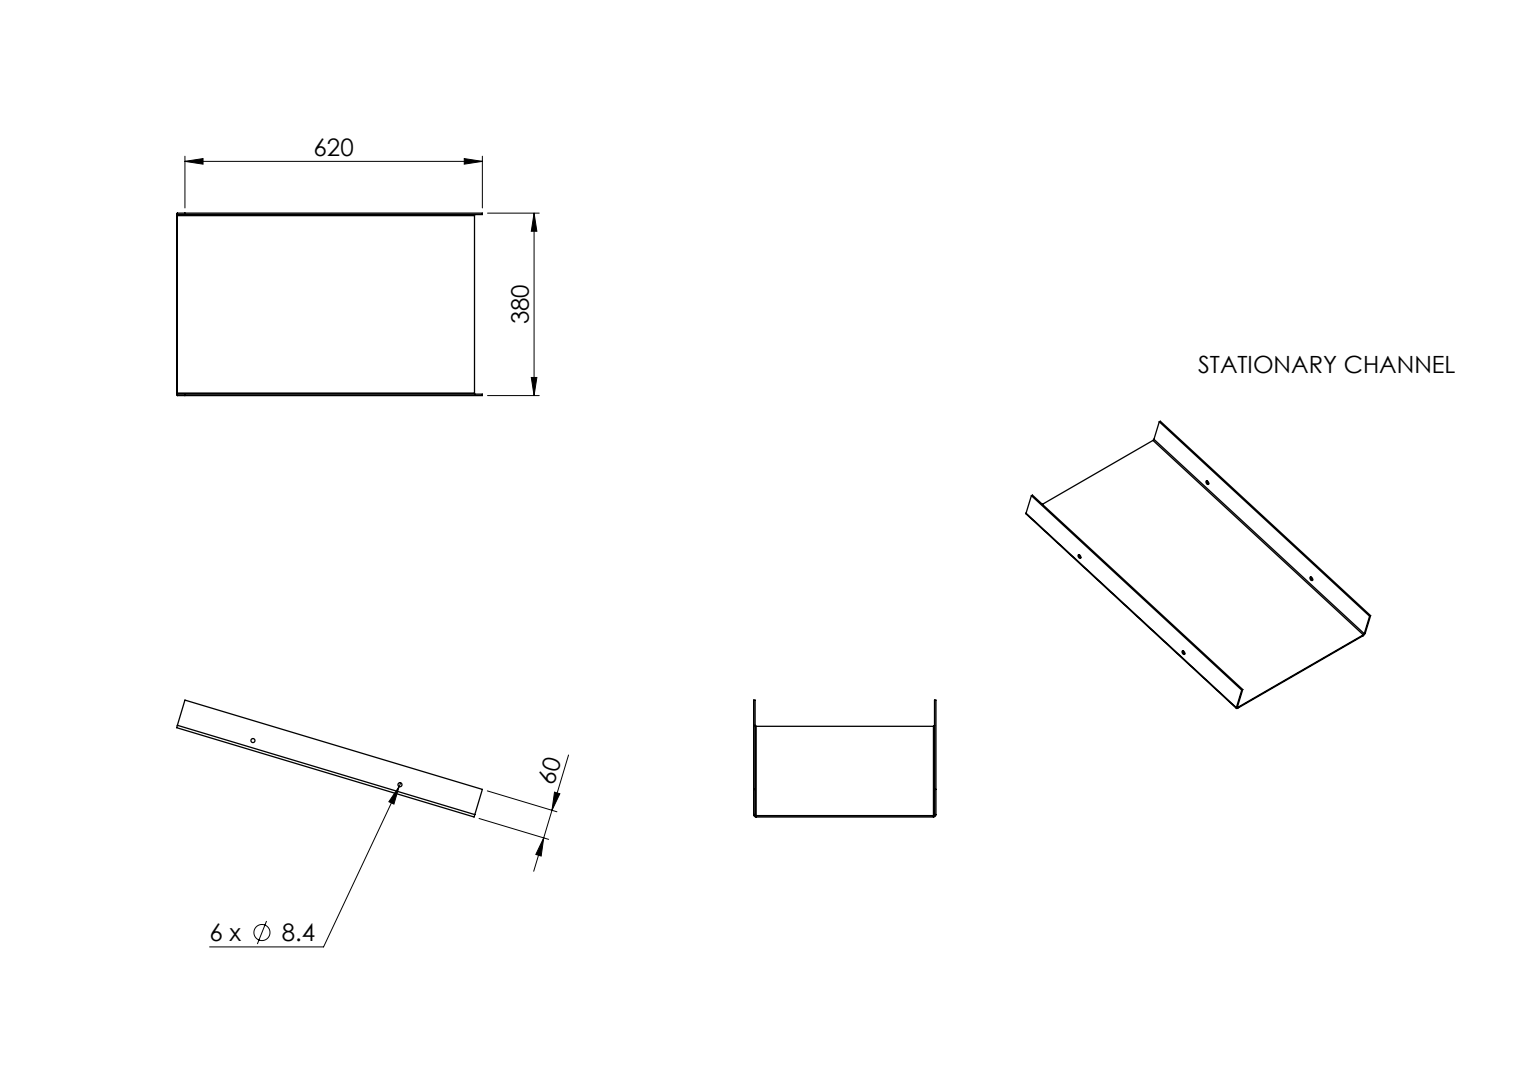
ISO-10303-21;
HEADER;
FILE_DESCRIPTION (('STEP AP214'),
    '1' );
FILE_NAME ('stationary channel.step',
    '2026-10-27T17:01:19',
    ( '' ),
    ( '' ),
    'SwSTEP 2.0',
    'SolidWorks 2026',
    '' );
FILE_SCHEMA (( 'AUTOMOTIVE_DESIGN' ));
ENDSEC;

DATA;
#27=FACE_OUTER_BOUND ( 'NONE', #636, .T. ) ;
#100=EDGE_LOOP ( 'NONE', ( #955, #2493 ) ) ;
#108=CARTESIAN_POINT ( 'NONE',  ( 610.0000000000000000, 227.4403065089097993, 184.7999999999999829 ) ) ;
#123=EDGE_CURVE ( 'NONE', #7138, #2816, #1501, .T. ) ;
#126=EDGE_CURVE ( 'NONE', #13510, #3531, #3853, .T. ) ;
#129=ORIENTED_EDGE ( 'NONE', *, *, #11764, .F. ) ;
#141=EDGE_CURVE ( 'NONE', #2225, #13547, #11826, .T. ) ;
#143=ORIENTED_EDGE ( 'NONE', *, *, #1858, .T. ) ;
#160=ADVANCED_FACE ( 'NONE', ( #9907 ), #3261, .F. ) ;
#164=ORIENTED_EDGE ( 'NONE', *, *, #10968, .F. ) ;
#185=PLANE ( 'NONE',  #4357 ) ;
#220=CIRCLE ( 'NONE', #10375, 2.199999999999988187 ) ;
#233=VECTOR ( 'NONE', #11079, 1000.000000000000000 ) ;
#245=CIRCLE ( 'NONE', #8768, 4.199999999999926459 ) ;
#249=DIRECTION ( 'NONE',  ( 0.9578262852211507639, -0.2873478855663477716, 0.000000000000000000 ) ) ;
#250=CARTESIAN_POINT ( 'NONE',  ( 153.1991633467111456, 386.6211705227183870, -210.0000000000000000 ) ) ;
#251=CARTESIAN_POINT ( 'NONE',  ( 627.2408731339806991, 284.9098836221797342, 190.0000000000001990 ) ) ;
#277=EDGE_LOOP ( 'NONE', ( #11682, #4913 ) ) ;
#280=LINE ( 'NONE', #3777, #11997 ) ;
#304=DIRECTION ( 'NONE',  ( 0.2873478855663427756, 0.9578262852211522071, 3.408579461568464094E-15 ) ) ;
#314=LINE ( 'NONE', #3891, #1590 ) ;
#379=VECTOR ( 'NONE', #7531, 1000.000000000000000 ) ;
#429=CARTESIAN_POINT ( 'NONE',  ( -8.505790995054768544, 418.4210031920615620, -184.7999999999999829 ) ) ;
#474=CARTESIAN_POINT ( 'NONE',  ( -9.137956343300835726, 416.3137853645748692, 184.7999999999999829 ) ) ;
#490=CARTESIAN_POINT ( 'NONE',  ( -1.861313246464723443E-13, -6.204377488215742287E-13, -186.9999999999986358 ) ) ;
#533=DIRECTION ( 'NONE',  ( -0.2873478855663454401, -0.9578262852211514300, -3.548540470164184620E-15 ) ) ;
#535=DIRECTION ( 'NONE',  ( -0.9578262852211513190, 0.2873478855663455511, 5.916456789157588541E-31 ) ) ;
#561=EDGE_CURVE ( 'NONE', #2165, #8693, #8490, .T. ) ;
#571=ORIENTED_EDGE ( 'NONE', *, *, #126, .T. ) ;
#576=DIRECTION ( 'NONE',  ( 0.9578262852211509859, -0.2873478855663466613, -4.622231866529364646E-30 ) ) ;
#588=DIRECTION ( 'NONE',  ( 9.794481010665704304E-16, 3.264827003555234768E-15, -1.000000000000000000 ) ) ;
#600=PLANE ( 'NONE',  #7043 ) ;
#605=ORIENTED_EDGE ( 'NONE', *, *, #2988, .F. ) ;
#610=LINE ( 'NONE', #474, #9375 ) ;
#626=DIRECTION ( 'NONE',  ( -0.9578262852211506528, 0.2873478855663477161, -0.000000000000000000 ) ) ;
#628=ORIENTED_EDGE ( 'NONE', *, *, #1225, .F. ) ;
#636=EDGE_LOOP ( 'NONE', ( #8796, #4569, #3020, #13957 ) ) ;
#679=CIRCLE ( 'NONE', #4453, 4.199999999999926459 ) ;
#681=VERTEX_POINT ( 'NONE', #2049 ) ;
#755=CARTESIAN_POINT ( 'NONE',  ( 153.1991633467111456, 386.6211705227183870, -190.0000000000000568 ) ) ;
#761=ORIENTED_EDGE ( 'NONE', *, *, #6990, .T. ) ;
#766=AXIS2_PLACEMENT_3D ( 'NONE', #3828, #7354, #8310 ) ;
#786=CARTESIAN_POINT ( 'NONE',  ( 451.3035746174797396, 294.6698471414878782, 190.0000000000000568 ) ) ;
#789=LINE ( 'NONE', #846, #1204 ) ;
#807=ADVANCED_FACE ( 'NONE', ( #7749 ), #14614, .F. ) ;
#812=ADVANCED_FACE ( 'NONE', ( #2126 ), #185, .T. ) ;
#820=DIRECTION ( 'NONE',  ( 0.000000000000000000, 1.000000000000000000, 0.000000000000000000 ) ) ;
#824=FACE_OUTER_BOUND ( 'NONE', #10572, .T. ) ;
#840=ORIENTED_EDGE ( 'NONE', *, *, #9284, .F. ) ;
#846=CARTESIAN_POINT ( 'NONE',  ( 610.8620436566989156, 230.3137853645742155, -187.0000000000000000 ) ) ;
#852=VERTEX_POINT ( 'NONE', #8038 ) ;
#858=DIRECTION ( 'NONE',  ( 0.2873478855663483267, 0.9578262852211505418, 0.000000000000000000 ) ) ;
#862=VECTOR ( 'NONE', #10859, 1000.000000000000114 ) ;
#863=CIRCLE ( 'NONE', #11005, 4.199999999999926459 ) ;
#868=DIRECTION ( 'NONE',  ( 1.921916333308140812E-15, 6.406387777693824270E-15, -1.000000000000000000 ) ) ;
#872=AXIS2_PLACEMENT_3D ( 'NONE', #1257, #4650, #7898 ) ;
#942=EDGE_CURVE ( 'NONE', #8737, #2165, #12678, .T. ) ;
#953=( GEOMETRIC_REPRESENTATION_CONTEXT ( 3 ) GLOBAL_UNCERTAINTY_ASSIGNED_CONTEXT ( ( #3993 ) ) GLOBAL_UNIT_ASSIGNED_CONTEXT ( ( #2035, #12214, #5452 ) ) REPRESENTATION_CONTEXT ( 'NONE', 'WORKASPACE' ) );
#955=ORIENTED_EDGE ( 'NONE', *, *, #1459, .T. ) ;
#958=DIRECTION ( 'NONE',  ( 0.000000000000000000, 1.000000000000000000, 3.264827003555234768E-15 ) ) ;
#985=ORIENTED_EDGE ( 'NONE', *, *, #1375, .T. ) ;
#995=AXIS2_PLACEMENT_3D ( 'NONE', #2091, #13260, #4330 ) ;
#1012=VERTEX_POINT ( 'NONE', #4251 ) ;
#1014=DIRECTION ( 'NONE',  ( 0.9578262852211507639, -0.2873478855663477716, 0.000000000000000000 ) ) ;
#1020=DIRECTION ( 'NONE',  ( -0.000000000000000000, -0.000000000000000000, -1.000000000000000000 ) ) ;
#1044=ADVANCED_FACE ( 'NONE', ( #2017 ), #14502, .F. ) ;
#1072=CARTESIAN_POINT ( 'NONE',  ( 455.5035746174796714, 294.6698471414878782, 187.0000000000000568 ) ) ;
#1131=ADVANCED_FACE ( 'NONE', ( #11459 ), #3428, .F. ) ;
#1141=AXIS2_PLACEMENT_3D ( 'NONE', #1241, #5744, #10241 ) ;
#1165=DIRECTION ( 'NONE',  ( 1.000000000000000000, 0.000000000000000000, 0.000000000000000000 ) ) ;
#1176=EDGE_LOOP ( 'NONE', ( #12389, #12490, #761, #12684 ) ) ;
#1178=CARTESIAN_POINT ( 'NONE',  ( 611.4942090049449916, 232.4210031920605388, 187.0000000000000000 ) ) ;
#1204=VECTOR ( 'NONE', #5366, 1000.000000000000227 ) ;
#1225=EDGE_CURVE ( 'NONE', #852, #13547, #7265, .T. ) ;
#1241=CARTESIAN_POINT ( 'NONE',  ( -8.505790995054995918, 418.4210031920614483, 184.7999999999999829 ) ) ;
#1247=AXIS2_PLACEMENT_3D ( 'NONE', #5486, #5271, #5189 ) ;
#1257=CARTESIAN_POINT ( 'NONE',  ( 611.4942090049451053, 232.4210031920599420, -184.7999999999999829 ) ) ;
#1274=CARTESIAN_POINT ( 'NONE',  ( 627.2408731339806991, 284.9098836221797342, 187.0000000000001990 ) ) ;
#1285=DIRECTION ( 'NONE',  ( -0.2873478855663483267, -0.9578262852211505418, -5.337610695313246651E-15 ) ) ;
#1318=DIRECTION ( 'NONE',  ( 0.9578262852211513190, -0.2873478855663453846, 0.000000000000000000 ) ) ;
#1333=EDGE_LOOP ( 'NONE', ( #7672, #14460, #2611, #6334 ) ) ;
#1344=LINE ( 'NONE', #4537, #4523 ) ;
#1347=EDGE_LOOP ( 'NONE', ( #7153, #12726, #8039, #8024 ) ) ;
#1354=DIRECTION ( 'NONE',  ( -0.2873478855663441633, -0.9578262852211516520, 3.408579461568462910E-15 ) ) ;
#1373=ORIENTED_EDGE ( 'NONE', *, *, #126, .F. ) ;
#1374=ADVANCED_FACE ( 'NONE', ( #4987 ), #9704, .F. ) ;
#1375=EDGE_CURVE ( 'NONE', #6946, #8693, #8587, .T. ) ;
#1376=VERTEX_POINT ( 'NONE', #755 ) ;
#1384=FACE_OUTER_BOUND ( 'NONE', #9975, .T. ) ;
#1390=CARTESIAN_POINT ( 'NONE',  ( 611.4942090049451053, 232.4210031920605388, 190.0000000000000000 ) ) ;
#1423=VECTOR ( 'NONE', #7760, 1000.000000000000000 ) ;
#1434=DIRECTION ( 'NONE',  ( -0.000000000000000000, -0.000000000000000000, 1.000000000000000000 ) ) ;
#1448=CIRCLE ( 'NONE', #1920, 4.199999999999926459 ) ;
#1459=EDGE_CURVE ( 'NONE', #10035, #14129, #8436, .T. ) ;
#1460=EDGE_LOOP ( 'NONE', ( #10013, #14172, #4888, #11929 ) ) ;
#1501=LINE ( 'NONE', #12864, #2181 ) ;
#1504=EDGE_CURVE ( 'NONE', #6153, #7939, #11006, .T. ) ;
#1516=LINE ( 'NONE', #9412, #9511 ) ;
#1526=EDGE_CURVE ( 'NONE', #10480, #13545, #3745, .T. ) ;
#1546=DIRECTION ( 'NONE',  ( -0.9578262852211507639, 0.2873478855663477716, -0.000000000000000000 ) ) ;
#1548=PLANE ( 'NONE',  #11567 ) ;
#1552=LINE ( 'NONE', #10711, #12900 ) ;
#1584=CARTESIAN_POINT ( 'NONE',  ( 611.4942090049448780, 232.4210031920598283, 184.7999999999999829 ) ) ;
#1590=VECTOR ( 'NONE', #9416, 1000.000000000000000 ) ;
#1592=VECTOR ( 'NONE', #10818, 1000.000000000000114 ) ;
#1596=DIRECTION ( 'NONE',  ( -0.000000000000000000, -0.000000000000000000, -1.000000000000000000 ) ) ;
#1618=FACE_BOUND ( 'NONE', #5385, .T. ) ;
#1633=FACE_BOUND ( 'NONE', #13457, .T. ) ;
#1648=DIRECTION ( 'NONE',  ( -0.2873478855663427756, -0.9578262852211522071, 0.000000000000000000 ) ) ;
#1702=AXIS2_PLACEMENT_3D ( 'NONE', #4505, #4645, #1165 ) ;
#1718=PLANE ( 'NONE',  #13443 ) ;
#1726=EDGE_CURVE ( 'NONE', #9048, #852, #1552, .T. ) ;
#1728=DIRECTION ( 'NONE',  ( 9.794481010665704304E-16, 3.264827003555234768E-15, -1.000000000000000000 ) ) ;
#1748=EDGE_CURVE ( 'NONE', #6946, #6153, #12852, .T. ) ;
#1756=ORIENTED_EDGE ( 'NONE', *, *, #1901, .F. ) ;
#1768=EDGE_LOOP ( 'NONE', ( #1792, #14548 ) ) ;
#1777=CARTESIAN_POINT ( 'NONE',  ( -10.00000000000007105, 413.4403065089107372, 184.7999999999999829 ) ) ;
#1792=ORIENTED_EDGE ( 'NONE', *, *, #10146, .T. ) ;
#1796=CARTESIAN_POINT ( 'NONE',  ( 610.8620436566991430, 230.3137853645733912, -184.7999999999999829 ) ) ;
#1802=LINE ( 'NONE', #11845, #13199 ) ;
#1847=CARTESIAN_POINT ( 'NONE',  ( 611.4942090049448780, 232.4210031920598283, 187.0000000000000000 ) ) ;
#1858=EDGE_CURVE ( 'NONE', #5524, #13510, #8711, .T. ) ;
#1869=EDGE_LOOP ( 'NONE', ( #5841, #9339, #9809, #5523 ) ) ;
#1870=ADVANCED_FACE ( 'NONE', ( #13141 ), #5390, .T. ) ;
#1901=EDGE_CURVE ( 'NONE', #4077, #8268, #9755, .T. ) ;
#1904=PRESENTATION_STYLE_ASSIGNMENT (( #3013 ) ) ;
#1912=VERTEX_POINT ( 'NONE', #14396 ) ;
#1916=DIRECTION ( 'NONE',  ( -0.000000000000000000, -0.000000000000000000, -1.000000000000000000 ) ) ;
#1920=AXIS2_PLACEMENT_3D ( 'NONE', #3888, #7564, #11017 ) ;
#1933=ADVANCED_FACE ( 'NONE', ( #6571 ), #14256, .F. ) ;
#1940=ORIENTED_EDGE ( 'NONE', *, *, #5847, .F. ) ;
#1961=LINE ( 'NONE', #10363, #9746 ) ;
#1966=EDGE_CURVE ( 'NONE', #7989, #9048, #9818, .T. ) ;
#1981=CARTESIAN_POINT ( 'NONE',  ( 611.4942090049451053, 232.4210031920599135, -187.0000000000000000 ) ) ;
#1987=DIRECTION ( 'NONE',  ( -1.000000000000000000, 0.000000000000000000, 0.000000000000000000 ) ) ;
#2007=CARTESIAN_POINT ( 'NONE',  ( 627.2408731339805854, 284.9098836221799615, -190.0000000000001990 ) ) ;
#2017=FACE_OUTER_BOUND ( 'NONE', #1333, .T. ) ;
#2027=EDGE_CURVE ( 'NONE', #4077, #13098, #3961, .T. ) ;
#2035=( LENGTH_UNIT ( ) NAMED_UNIT ( * ) SI_UNIT ( .MILLI., .METRE. ) );
#2041=ADVANCED_FACE ( 'NONE', ( #3327 ), #8042, .T. ) ;
#2044=AXIS2_PLACEMENT_3D ( 'NONE', #7770, #12258, #820 ) ;
#2049=CARTESIAN_POINT ( 'NONE',  ( 610.8620436566989156, 230.3137853645732775, 184.7999999999999829 ) ) ;
#2055=DIRECTION ( 'NONE',  ( 0.000000000000000000, -1.000000000000000000, 0.000000000000000000 ) ) ;
#2065=AXIS2_PLACEMENT_3D ( 'NONE', #9984, #3195, #2069 ) ;
#2069=DIRECTION ( 'NONE',  ( 0.000000000000000000, -1.000000000000000000, 0.000000000000000000 ) ) ;
#2091=CARTESIAN_POINT ( 'NONE',  ( 148.9991633467111569, 386.6211705227183870, -187.0000000000000568 ) ) ;
#2096=CARTESIAN_POINT ( 'NONE',  ( -8.505790995054976378, 418.4210031920615052, 190.0000000000000000 ) ) ;
#2107=DIRECTION ( 'NONE',  ( -0.2873478855663396114, -0.9578262852211530953, 0.000000000000000000 ) ) ;
#2125=VECTOR ( 'NONE', #7691, 1000.000000000000000 ) ;
#2126=FACE_OUTER_BOUND ( 'NONE', #7480, .T. ) ;
#2143=AXIS2_PLACEMENT_3D ( 'NONE', #9097, #2226, #2158 ) ;
#2149=ORIENTED_EDGE ( 'NONE', *, *, #13921, .T. ) ;
#2154=CIRCLE ( 'NONE', #12535, 2.199999999999988187 ) ;
#2158=DIRECTION ( 'NONE',  ( -1.000000000000000000, 0.000000000000000000, 0.000000000000000000 ) ) ;
#2165=VERTEX_POINT ( 'NONE', #10406 ) ;
#2181=VECTOR ( 'NONE', #8424, 1000.000000000000000 ) ;
#2198=FACE_BOUND ( 'NONE', #8661, .T. ) ;
#2201=FACE_OUTER_BOUND ( 'NONE', #14284, .T. ) ;
#2220=ORIENTED_EDGE ( 'NONE', *, *, #11012, .T. ) ;
#2225=VERTEX_POINT ( 'NONE', #1981 ) ;
#2226=DIRECTION ( 'NONE',  ( -0.000000000000000000, -0.000000000000000000, -1.000000000000000000 ) ) ;
#2248=SHAPE_REPRESENTATION ( 'stationary channel', ( #9440 ), #8508 ) ;
#2274=ORIENTED_EDGE ( 'NONE', *, *, #942, .T. ) ;
#2275=ORIENTED_EDGE ( 'NONE', *, *, #9049, .T. ) ;
#2288=EDGE_CURVE ( 'NONE', #12648, #9517, #610, .T. ) ;
#2304=DIRECTION ( 'NONE',  ( -0.000000000000000000, -0.000000000000000000, 1.000000000000000000 ) ) ;
#2307=EDGE_CURVE ( 'NONE', #10292, #10447, #314, .T. ) ;
#2320=VECTOR ( 'NONE', #13632, 1000.000000000000227 ) ;
#2325=CARTESIAN_POINT ( 'NONE',  ( -122.9652219749294488, 36.88956659247806869, -189.9999999999986358 ) ) ;
#2342=PLANE ( 'NONE',  #11572 ) ;
#2348=CARTESIAN_POINT ( 'NONE',  ( 112.9652219749295483, 376.5507399164318372, 1.650218294979717018E-14 ) ) ;
#2350=DIRECTION ( 'NONE',  ( -0.2873478855663477716, -0.9578262852211506528, 0.000000000000000000 ) ) ;
#2406=DIRECTION ( 'NONE',  ( -9.794481010665704304E-16, -3.264827003555233190E-15, -1.000000000000000000 ) ) ;
#2413=DIRECTION ( 'NONE',  ( 0.2873478855663448850, 0.9578262852211515410, -3.408579461568462910E-15 ) ) ;
#2416=VECTOR ( 'NONE', #6630, 1000.000000000000000 ) ;
#2424=( GEOMETRIC_REPRESENTATION_CONTEXT ( 3 ) GLOBAL_UNCERTAINTY_ASSIGNED_CONTEXT ( ( #13447 ) ) GLOBAL_UNIT_ASSIGNED_CONTEXT ( ( #2705, #7205, #13845 ) ) REPRESENTATION_CONTEXT ( 'NONE', 'WORKASPACE' ) );
#2428=DIRECTION ( 'NONE',  ( 0.2873478855663454401, 0.9578262852211513190, 0.000000000000000000 ) ) ;
#2438=ORIENTED_EDGE ( 'NONE', *, *, #10439, .T. ) ;
#2493=ORIENTED_EDGE ( 'NONE', *, *, #12109, .T. ) ;
#2500=VERTEX_POINT ( 'NONE', #1847 ) ;
#2505=PRODUCT_DEFINITION_SHAPE ( 'NONE', 'NONE',  #5588 ) ;
#2524=AXIS2_PLACEMENT_3D ( 'NONE', #14594, #3384, #7942 ) ;
#2549=AXIS2_PLACEMENT_3D ( 'NONE', #12721, #11396, #1285 ) ;
#2589=LINE ( 'NONE', #3410, #5681 ) ;
#2611=ORIENTED_EDGE ( 'NONE', *, *, #123, .T. ) ;
#2631=CIRCLE ( 'NONE', #12512, 4.199999999999981526 ) ;
#2661=ORIENTED_EDGE ( 'NONE', *, *, #1966, .F. ) ;
#2665=LINE ( 'NONE', #6881, #11080 ) ;
#2672=CARTESIAN_POINT ( 'NONE',  ( 497.0347780250717733, -149.1104334075207589, 189.9999999999986358 ) ) ;
#2705=( LENGTH_UNIT ( ) NAMED_UNIT ( * ) SI_UNIT ( .MILLI., .METRE. ) );
#2744=ORIENTED_EDGE ( 'NONE', *, *, #2027, .F. ) ;
#2745=DIRECTION ( 'NONE',  ( -0.2873478855663480491, -0.9578262852211507639, 0.000000000000000000 ) ) ;
#2782=CYLINDRICAL_SURFACE ( 'NONE', #3577, 4.199999999999981526 ) ;
#2793=ORIENTED_EDGE ( 'NONE', *, *, #9284, .T. ) ;
#2816=VERTEX_POINT ( 'NONE', #8845 ) ;
#2827=LINE ( 'NONE', #13427, #5208 ) ;
#2833=EDGE_CURVE ( 'NONE', #6946, #8674, #3743, .T. ) ;
#2852=CYLINDRICAL_SURFACE ( 'NONE', #766, 2.200000000000007283 ) ;
#2865=LINE ( 'NONE', #3837, #14610 ) ;
#2894=ORIENTED_EDGE ( 'NONE', *, *, #14304, .T. ) ;
#2902=VERTEX_POINT ( 'NONE', #11482 ) ;
#2913=CARTESIAN_POINT ( 'NONE',  ( 627.2408731339806991, 284.9098836221797342, 190.0000000000001990 ) ) ;
#2929=CARTESIAN_POINT ( 'NONE',  ( -122.9652219749301736, 36.88956659247854475, 189.9999999999986358 ) ) ;
#2943=( NAMED_UNIT ( * ) SI_UNIT ( $, .STERADIAN. ) SOLID_ANGLE_UNIT ( ) );
#2960=DIRECTION ( 'NONE',  ( -0.2873478855663454401, -0.9578262852211513190, 0.000000000000000000 ) ) ;
#2977=CARTESIAN_POINT ( 'NONE',  ( 455.5035746174796714, 294.6698471414878782, 190.0000000000000568 ) ) ;
#2984=ORIENTED_EDGE ( 'NONE', *, *, #3700, .T. ) ;
#2988=EDGE_CURVE ( 'NONE', #9517, #8693, #12207, .T. ) ;
#3002=EDGE_CURVE ( 'NONE', #10447, #9874, #8027, .T. ) ;
#3013=SURFACE_STYLE_USAGE ( .BOTH. , #13122 ) ;
#3020=ORIENTED_EDGE ( 'NONE', *, *, #5314, .T. ) ;
#3026=CARTESIAN_POINT ( 'NONE',  ( 7.240873133980807452, 470.9098836221798479, -190.0000000000001990 ) ) ;
#3032=CARTESIAN_POINT ( 'NONE',  ( 459.7035746174795463, 294.6698471414878782, 210.0000000000000000 ) ) ;
#3035=ADVANCED_FACE ( 'NONE', ( #11563, #8540, #12971 ), #9923, .T. ) ;
#3038=ORIENTED_EDGE ( 'NONE', *, *, #10054, .T. ) ;
#3050=ORIENTED_EDGE ( 'NONE', *, *, #6990, .F. ) ;
#3052=DIRECTION ( 'NONE',  ( -0.2873478855663441633, -0.9578262852211516520, 0.000000000000000000 ) ) ;
#3088=STYLED_ITEM ( 'NONE', ( #1904 ), #12520 ) ;
#3101=DIRECTION ( 'NONE',  ( 0.000000000000000000, -1.000000000000000000, 3.264827003555233190E-15 ) ) ;
#3167=( NAMED_UNIT ( * ) PLANE_ANGLE_UNIT ( ) SI_UNIT ( $, .RADIAN. ) );
#3194=ORIENTED_EDGE ( 'NONE', *, *, #6816, .T. ) ;
#3195=DIRECTION ( 'NONE',  ( -9.794481010665704304E-16, -3.264827003555233190E-15, -1.000000000000000000 ) ) ;
#3223=VERTEX_POINT ( 'NONE', #3421 ) ;
#3228=SHAPE_REPRESENTATION_RELATIONSHIP ( 'NONE' , 'NONE' ,  #2248, #12520 ) ;
#3233=CARTESIAN_POINT ( 'NONE',  ( 611.4942090049448780, 232.4210031920598283, 184.7999999999999829 ) ) ;
#3261=PLANE ( 'NONE',  #1247 ) ;
#3270=AXIS2_PLACEMENT_3D ( 'NONE', #12259, #6671, #4530 ) ;
#3276=ORIENTED_EDGE ( 'NONE', *, *, #8006, .T. ) ;
#3298=EDGE_LOOP ( 'NONE', ( #3194, #14214 ) ) ;
#3299=DIRECTION ( 'NONE',  ( 0.000000000000000000, 1.000000000000000000, 0.000000000000000000 ) ) ;
#3327=FACE_OUTER_BOUND ( 'NONE', #14566, .T. ) ;
#3344=LINE ( 'NONE', #5545, #2125 ) ;
#3351=CIRCLE ( 'NONE', #7344, 2.200000000000009948 ) ;
#3384=DIRECTION ( 'NONE',  ( -0.9578262852211507639, 0.2873478855663477716, 0.000000000000000000 ) ) ;
#3406=DIRECTION ( 'NONE',  ( -0.9578262852211507639, 0.2873478855663477716, 0.000000000000000000 ) ) ;
#3410=CARTESIAN_POINT ( 'NONE',  ( -9.999999999999840128, 413.4403065089115330, -184.7999999999999829 ) ) ;
#3421=CARTESIAN_POINT ( 'NONE',  ( 144.7991633467111683, 386.6211705227183870, 190.0000000000000568 ) ) ;
#3422=DIRECTION ( 'NONE',  ( 0.2873478855663477161, 0.9578262852211506528, 0.000000000000000000 ) ) ;
#3428=CYLINDRICAL_SURFACE ( 'NONE', #4683, 4.199999999999926459 ) ;
#3443=CYLINDRICAL_SURFACE ( 'NONE', #2524, 2.200000000000007283 ) ;
#3450=ORIENTED_EDGE ( 'NONE', *, *, #12173, .F. ) ;
#3462=LINE ( 'NONE', #11427, #6116 ) ;
#3502=VERTEX_POINT ( 'NONE', #7543 ) ;
#3506=VECTOR ( 'NONE', #11881, 1000.000000000000114 ) ;
#3531=VERTEX_POINT ( 'NONE', #9693 ) ;
#3547=ORIENTED_EDGE ( 'NONE', *, *, #10808, .F. ) ;
#3573=FACE_OUTER_BOUND ( 'NONE', #6762, .T. ) ;
#3577=AXIS2_PLACEMENT_3D ( 'NONE', #12000, #1596, #7364 ) ;
#3588=FACE_OUTER_BOUND ( 'NONE', #6490, .T. ) ;
#3619=CARTESIAN_POINT ( 'NONE',  ( 148.9991633467111569, 386.6211705227183870, 187.0000000000000568 ) ) ;
#3626=CARTESIAN_POINT ( 'NONE',  ( 451.3035746174797396, 294.6698471414878782, 187.0000000000000568 ) ) ;
#3668=DIRECTION ( 'NONE',  ( 0.9578262852211513190, -0.2873478855663453846, 0.000000000000000000 ) ) ;
#3677=ORIENTED_EDGE ( 'NONE', *, *, #13247, .F. ) ;
#3700=EDGE_CURVE ( 'NONE', #9517, #3531, #280, .T. ) ;
#3743=CIRCLE ( 'NONE', #13633, 5.200000000000005507 ) ;
#3745=CIRCLE ( 'NONE', #2044, 4.199999999999981526 ) ;
#3757=ORIENTED_EDGE ( 'NONE', *, *, #141, .T. ) ;
#3777=CARTESIAN_POINT ( 'NONE',  ( -9.999999999999980460, 413.4403065089106235, 190.0000000000000000 ) ) ;
#3790=VECTOR ( 'NONE', #9846, 1000.000000000000000 ) ;
#3828=CARTESIAN_POINT ( 'NONE',  ( 611.4942090049449916, 232.4210031920597999, 184.7999999999999829 ) ) ;
#3837=CARTESIAN_POINT ( 'NONE',  ( 610.8620436566990293, 230.3137853645732491, 184.7999999999999829 ) ) ;
#3850=ORIENTED_EDGE ( 'NONE', *, *, #14304, .F. ) ;
#3853=CIRCLE ( 'NONE', #5726, 5.200000000000004619 ) ;
#3888=CARTESIAN_POINT ( 'NONE',  ( 455.5035746174796714, 294.6698471414878782, -190.0000000000000568 ) ) ;
#3891=CARTESIAN_POINT ( 'NONE',  ( 7.240873133980807452, 470.9098836221799047, -190.0000000000001990 ) ) ;
#3893=CARTESIAN_POINT ( 'NONE',  ( 459.7035746174795463, 294.6698471414878782, -210.0000000000000000 ) ) ;
#3894=DIRECTION ( 'NONE',  ( -0.000000000000000000, -0.000000000000000000, -1.000000000000000000 ) ) ;
#3909=DIRECTION ( 'NONE',  ( 0.000000000000000000, -1.000000000000000000, 0.000000000000000000 ) ) ;
#3920=ADVANCED_FACE ( 'NONE', ( #1618, #7521, #3987 ), #12915, .F. ) ;
#3924=DIRECTION ( 'NONE',  ( -0.2873478855663894049, -0.9578262852211382183, 0.000000000000000000 ) ) ;
#3948=ADVANCED_FACE ( 'NONE', ( #2198, #4417, #13344 ), #6562, .F. ) ;
#3955=DIRECTION ( 'NONE',  ( 0.000000000000000000, -5.337610695313242707E-15, 1.000000000000000000 ) ) ;
#3961=CIRCLE ( 'NONE', #11019, 4.199999999999926459 ) ;
#3971=CARTESIAN_POINT ( 'NONE',  ( -8.505790995054773873, 418.4210031920615620, -187.0000000000000000 ) ) ;
#3987=FACE_OUTER_BOUND ( 'NONE', #13183, .T. ) ;
#3993=UNCERTAINTY_MEASURE_WITH_UNIT (LENGTH_MEASURE( 1.000000000000000082E-05 ), #2035, 'distance_accuracy_value', 'NONE');
#4024=ORIENTED_EDGE ( 'NONE', *, *, #8205, .F. ) ;
#4036=CARTESIAN_POINT ( 'NONE',  ( 153.1991633467111456, 386.6211705227183870, 190.0000000000000568 ) ) ;
#4062=AXIS2_PLACEMENT_3D ( 'NONE', #13779, #4922, #3668 ) ;
#4077=VERTEX_POINT ( 'NONE', #11202 ) ;
#4085=VERTEX_POINT ( 'NONE', #14387 ) ;
#4101=DIRECTION ( 'NONE',  ( -0.9578262852211522071, 0.2873478855663427756, -9.629649721936179265E-30 ) ) ;
#4119=DIRECTION ( 'NONE',  ( 9.794481010665704304E-16, 3.264827003555234768E-15, -1.000000000000000000 ) ) ;
#4155=DIRECTION ( 'NONE',  ( -0.9578262852211513190, 0.2873478855663453846, 0.000000000000000000 ) ) ;
#4203=AXIS2_PLACEMENT_3D ( 'NONE', #8824, #8470, #8883 ) ;
#4232=EDGE_CURVE ( 'NONE', #681, #12648, #2865, .T. ) ;
#4251=CARTESIAN_POINT ( 'NONE',  ( 459.7035746174795463, 294.6698471414878782, -190.0000000000000568 ) ) ;
#4330=DIRECTION ( 'NONE',  ( 0.000000000000000000, -1.000000000000000000, 0.000000000000000000 ) ) ;
#4346=LINE ( 'NONE', #7593, #2416 ) ;
#4347=CARTESIAN_POINT ( 'NONE',  ( 0.000000000000000000, 0.000000000000000000, 0.000000000000000000 ) ) ;
#4357=AXIS2_PLACEMENT_3D ( 'NONE', #2348, #5533, #1318 ) ;
#4367=ORIENTED_EDGE ( 'NONE', *, *, #1726, .F. ) ;
#4380=EDGE_LOOP ( 'NONE', ( #3757, #3450, #5668, #10845 ) ) ;
#4396=ORIENTED_EDGE ( 'NONE', *, *, #7209, .T. ) ;
#4399=ORIENTED_EDGE ( 'NONE', *, *, #11764, .T. ) ;
#4417=FACE_BOUND ( 'NONE', #277, .T. ) ;
#4453=AXIS2_PLACEMENT_3D ( 'NONE', #9724, #4119, #11992 ) ;
#4461=AXIS2_PLACEMENT_3D ( 'NONE', #13419, #10023, #3101 ) ;
#4505=CARTESIAN_POINT ( 'NONE',  ( 148.9991633467111569, 386.6211705227183870, 210.0000000000000000 ) ) ;
#4520=FACE_OUTER_BOUND ( 'NONE', #1347, .T. ) ;
#4523=VECTOR ( 'NONE', #8951, 1000.000000000000000 ) ;
#4530=DIRECTION ( 'NONE',  ( 0.000000000000000000, 1.000000000000000000, 0.000000000000000000 ) ) ;
#4537=CARTESIAN_POINT ( 'NONE',  ( 451.3035746174797396, 294.6698471414878782, 210.0000000000000000 ) ) ;
#4549=CARTESIAN_POINT ( 'NONE',  ( 455.5035746174796714, 294.6698471414878782, 210.0000000000000000 ) ) ;
#4569=ORIENTED_EDGE ( 'NONE', *, *, #11840, .T. ) ;
#4577=DIRECTION ( 'NONE',  ( 9.794481010665704304E-16, 3.264827003555234768E-15, -1.000000000000000000 ) ) ;
#4641=CARTESIAN_POINT ( 'NONE',  ( 627.2408731339805854, 284.9098836221799615, -187.0000000000001990 ) ) ;
#4644=FACE_OUTER_BOUND ( 'NONE', #12280, .T. ) ;
#4645=DIRECTION ( 'NONE',  ( -0.000000000000000000, -0.000000000000000000, 1.000000000000000000 ) ) ;
#4650=DIRECTION ( 'NONE',  ( 0.9578262852211507639, -0.2873478855663477716, -0.000000000000000000 ) ) ;
#4669=EDGE_LOOP ( 'NONE', ( #2744, #3547 ) ) ;
#4675=ORIENTED_EDGE ( 'NONE', *, *, #4232, .F. ) ;
#4683=AXIS2_PLACEMENT_3D ( 'NONE', #13828, #1434, #10286 ) ;
#4707=ORIENTED_EDGE ( 'NONE', *, *, #10439, .F. ) ;
#4726=DIRECTION ( 'NONE',  ( 0.9578262852211514300, -0.2873478855663454956, 0.000000000000000000 ) ) ;
#4768=EDGE_CURVE ( 'NONE', #10480, #3223, #1516, .T. ) ;
#4796=CARTESIAN_POINT ( 'NONE',  ( -8.505790995055013681, 418.4210031920606525, 187.0000000000000000 ) ) ;
#4811=CARTESIAN_POINT ( 'NONE',  ( 610.8620436566989156, 230.3137853645732775, 184.7999999999999829 ) ) ;
#4815=ORIENTED_EDGE ( 'NONE', *, *, #942, .F. ) ;
#4847=EDGE_CURVE ( 'NONE', #5524, #10447, #8525, .T. ) ;
#4880=ORIENTED_EDGE ( 'NONE', *, *, #1526, .T. ) ;
#4888=ORIENTED_EDGE ( 'NONE', *, *, #2307, .F. ) ;
#4902=VECTOR ( 'NONE', #6314, 1000.000000000000114 ) ;
#4913=ORIENTED_EDGE ( 'NONE', *, *, #10628, .T. ) ;
#4922=DIRECTION ( 'NONE',  ( -0.2873478855663454401, -0.9578262852211514300, -4.197634718856730240E-17 ) ) ;
#4978=CIRCLE ( 'NONE', #13216, 4.199999999999981526 ) ;
#4987=FACE_OUTER_BOUND ( 'NONE', #11240, .T. ) ;
#5004=DIRECTION ( 'NONE',  ( -0.2873478855662898734, -0.9578262852211680833, 0.000000000000000000 ) ) ;
#5039=ADVANCED_FACE ( 'NONE', ( #5710 ), #1548, .F. ) ;
#5075=FACE_OUTER_BOUND ( 'NONE', #11435, .T. ) ;
#5101=DIRECTION ( 'NONE',  ( 0.000000000000000000, -1.000000000000000000, 0.000000000000000000 ) ) ;
#5132=ADVANCED_FACE ( 'NONE', ( #11933 ), #9814, .F. ) ;
#5140=LINE ( 'NONE', #8531, #4902 ) ;
#5142=ADVANCED_FACE ( 'NONE', ( #9593 ), #9750, .F. ) ;
#5152=ORIENTED_EDGE ( 'NONE', *, *, #9828, .T. ) ;
#5168=AXIS2_PLACEMENT_3D ( 'NONE', #2977, #1728, #13023 ) ;
#5178=CARTESIAN_POINT ( 'NONE',  ( 459.7035746174795463, 294.6698471414878782, 190.0000000000000568 ) ) ;
#5180=ORIENTED_EDGE ( 'NONE', *, *, #3002, .F. ) ;
#5189=DIRECTION ( 'NONE',  ( -0.2873478855663477161, -0.9578262852211506528, 0.000000000000000000 ) ) ;
#5208=VECTOR ( 'NONE', #1020, 1000.000000000000000 ) ;
#5254=DIRECTION ( 'NONE',  ( 0.000000000000000000, 1.000000000000000000, 0.000000000000000000 ) ) ;
#5258=DIRECTION ( 'NONE',  ( 0.2873478855663448850, 0.9578262852211515410, 0.000000000000000000 ) ) ;
#5271=DIRECTION ( 'NONE',  ( -0.9578262852211507639, 0.2873478855663477716, 0.000000000000000000 ) ) ;
#5291=LINE ( 'NONE', #2929, #1592 ) ;
#5314=EDGE_CURVE ( 'NONE', #2225, #5524, #13857, .T. ) ;
#5322=CARTESIAN_POINT ( 'NONE',  ( -9.137956343300796647, 416.3137853645750397, -184.7999999999999829 ) ) ;
#5366=DIRECTION ( 'NONE',  ( -0.2873478855663441633, -0.9578262852211516520, 3.408579461568462910E-15 ) ) ;
#5385=EDGE_LOOP ( 'NONE', ( #7964, #2438 ) ) ;
#5390=PLANE ( 'NONE',  #8203 ) ;
#5414=VERTEX_POINT ( 'NONE', #786 ) ;
#5423=ADVANCED_FACE ( 'NONE', ( #7434 ), #2782, .F. ) ;
#5452=( NAMED_UNIT ( * ) SI_UNIT ( $, .STERADIAN. ) SOLID_ANGLE_UNIT ( ) );
#5470=DIRECTION ( 'NONE',  ( -0.9578262852211514300, 0.2873478855663454956, -1.399211572952243085E-16 ) ) ;
#5485=CIRCLE ( 'NONE', #995, 4.199999999999981526 ) ;
#5486=CARTESIAN_POINT ( 'NONE',  ( 611.4942090049448780, 232.4210031920598283, 184.7999999999999829 ) ) ;
#5510=ORIENTED_EDGE ( 'NONE', *, *, #141, .F. ) ;
#5521=DIRECTION ( 'NONE',  ( 0.9578262852211507639, -0.2873478855663477716, -0.000000000000000000 ) ) ;
#5523=ORIENTED_EDGE ( 'NONE', *, *, #12173, .T. ) ;
#5524=VERTEX_POINT ( 'NONE', #3971 ) ;
#5533=DIRECTION ( 'NONE',  ( -0.2873478855663454401, -0.9578262852211514300, -4.197634718856730240E-17 ) ) ;
#5535=CARTESIAN_POINT ( 'NONE',  ( -9.137956343300944084, 416.3137853645740734, 190.0000000000000000 ) ) ;
#5545=CARTESIAN_POINT ( 'NONE',  ( -9.137956343300944084, 416.3137853645740734, 190.0000000000000000 ) ) ;
#5566=CYLINDRICAL_SURFACE ( 'NONE', #7145, 4.199999999999926459 ) ;
#5585=LINE ( 'NONE', #4796, #12004 ) ;
#5588=PRODUCT_DEFINITION ( 'UNKNOWN', '', #13981, #6159 ) ;
#5651=VECTOR ( 'NONE', #3894, 1000.000000000000000 ) ;
#5656=VECTOR ( 'NONE', #10953, 1000.000000000000000 ) ;
#5665=VECTOR ( 'NONE', #11280, 1000.000000000000114 ) ;
#5668=ORIENTED_EDGE ( 'NONE', *, *, #9890, .T. ) ;
#5681=VECTOR ( 'NONE', #11510, 1000.000000000000114 ) ;
#5700=ORIENTED_EDGE ( 'NONE', *, *, #123, .F. ) ;
#5710=FACE_OUTER_BOUND ( 'NONE', #10408, .T. ) ;
#5726=AXIS2_PLACEMENT_3D ( 'NONE', #6000, #12937, #2745 ) ;
#5744=DIRECTION ( 'NONE',  ( -0.9578262852211507639, 0.2873478855663477716, -0.000000000000000000 ) ) ;
#5760=EDGE_LOOP ( 'NONE', ( #164, #9742, #13383, #11176 ) ) ;
#5790=ORIENTED_EDGE ( 'NONE', *, *, #10511, .T. ) ;
#5811=CARTESIAN_POINT ( 'NONE',  ( 7.240873133980769261, 470.9098836221799047, -187.0000000000001990 ) ) ;
#5827=DIRECTION ( 'NONE',  ( 1.460819769243627131E-16, 0.000000000000000000, -1.000000000000000000 ) ) ;
#5841=ORIENTED_EDGE ( 'NONE', *, *, #6407, .F. ) ;
#5847=EDGE_CURVE ( 'NONE', #2902, #7138, #863, .T. ) ;
#5848=ORIENTED_EDGE ( 'NONE', *, *, #10511, .F. ) ;
#5924=CIRCLE ( 'NONE', #7101, 4.199999999999981526 ) ;
#5937=PLANE ( 'NONE',  #8776 ) ;
#5946=ORIENTED_EDGE ( 'NONE', *, *, #10054, .F. ) ;
#5970=CARTESIAN_POINT ( 'NONE',  ( 455.5035746174796714, 294.6698471414878782, -190.0000000000000568 ) ) ;
#6000=CARTESIAN_POINT ( 'NONE',  ( -8.505790995054779202, 418.4210031920615620, -184.7999999999999829 ) ) ;
#6058=AXIS2_PLACEMENT_3D ( 'NONE', #14186, #6502, #5258 ) ;
#6116=VECTOR ( 'NONE', #2350, 1000.000000000000114 ) ;
#6153=VERTEX_POINT ( 'NONE', #251 ) ;
#6158=CARTESIAN_POINT ( 'NONE',  ( -8.505790995055013681, 418.4210031920606525, 190.0000000000000000 ) ) ;
#6159=PRODUCT_DEFINITION_CONTEXT ( 'detailed design', #10364, 'design' ) ;
#6160=LINE ( 'NONE', #10662, #6305 ) ;
#6250=ADVANCED_FACE ( 'NONE', ( #27 ), #3443, .F. ) ;
#6255=DIRECTION ( 'NONE',  ( 9.794481010665704304E-16, 3.264827003555233190E-15, 1.000000000000000000 ) ) ;
#6263=EDGE_CURVE ( 'NONE', #13510, #10292, #12437, .T. ) ;
#6299=ORIENTED_EDGE ( 'NONE', *, *, #1225, .T. ) ;
#6305=VECTOR ( 'NONE', #304, 1000.000000000000114 ) ;
#6314=DIRECTION ( 'NONE',  ( 0.9578262852211513190, -0.2873478855663455511, 1.972152263052529951E-31 ) ) ;
#6333=FILL_AREA_STYLE_COLOUR ( '', #7810 ) ;
#6334=ORIENTED_EDGE ( 'NONE', *, *, #10628, .F. ) ;
#6383=AXIS2_PLACEMENT_3D ( 'NONE', #11219, #3406, #7906 ) ;
#6401=EDGE_CURVE ( 'NONE', #4085, #8693, #5291, .T. ) ;
#6407=EDGE_CURVE ( 'NONE', #13510, #13547, #5140, .T. ) ;
#6417=DIRECTION ( 'NONE',  ( 1.000000000000000000, 0.000000000000000000, 0.000000000000000000 ) ) ;
#6426=CARTESIAN_POINT ( 'NONE',  ( -1.891179505616666007E-13, -6.303931685388887194E-13, 189.9999999999986358 ) ) ;
#6428=CARTESIAN_POINT ( 'NONE',  ( -9.137956343300963624, 416.3137853645741302, 190.0000000000000000 ) ) ;
#6446=EDGE_CURVE ( 'NONE', #10292, #1912, #13321, .T. ) ;
#6455=DIRECTION ( 'NONE',  ( 1.019665600948283447E-15, 3.398885336494278419E-15, -1.000000000000000000 ) ) ;
#6459=DIRECTION ( 'NONE',  ( 0.9578262852211513190, -0.2873478855663454401, 0.000000000000000000 ) ) ;
#6489=( LENGTH_UNIT ( ) NAMED_UNIT ( * ) SI_UNIT ( .MILLI., .METRE. ) );
#6490=EDGE_LOOP ( 'NONE', ( #840, #11714, #13876, #3677 ) ) ;
#6498=UNCERTAINTY_MEASURE_WITH_UNIT (LENGTH_MEASURE( 1.000000000000000082E-05 ), #6489, 'distance_accuracy_value', 'NONE');
#6502=DIRECTION ( 'NONE',  ( 0.9578262852211515410, -0.2873478855663448850, -2.182720603638867417E-30 ) ) ;
#6522=DIRECTION ( 'NONE',  ( -0.2873478855663454956, -0.9578262852211514300, 3.467246277775659127E-15 ) ) ;
#6523=EDGE_LOOP ( 'NONE', ( #13139, #4880, #4399, #4707 ) ) ;
#6562=PLANE ( 'NONE',  #4461 ) ;
#6566=CYLINDRICAL_SURFACE ( 'NONE', #8538, 5.200000000000009948 ) ;
#6571=FACE_OUTER_BOUND ( 'NONE', #1460, .T. ) ;
#6595=ORIENTED_EDGE ( 'NONE', *, *, #1459, .F. ) ;
#6630=DIRECTION ( 'NONE',  ( -0.000000000000000000, -0.000000000000000000, 1.000000000000000000 ) ) ;
#6663=ORIENTED_EDGE ( 'NONE', *, *, #12675, .F. ) ;
#6671=DIRECTION ( 'NONE',  ( 9.794481010665704304E-16, 3.264827003555234768E-15, -1.000000000000000000 ) ) ;
#6686=DIRECTION ( 'NONE',  ( 1.000000000000000000, 0.000000000000000000, 0.000000000000000000 ) ) ;
#6759=EDGE_CURVE ( 'NONE', #2500, #7939, #6160, .T. ) ;
#6762=EDGE_LOOP ( 'NONE', ( #12936, #6595, #2894, #4024 ) ) ;
#6816=EDGE_CURVE ( 'NONE', #8268, #5414, #12704, .T. ) ;
#6841=ADVANCED_FACE ( 'NONE', ( #14420 ), #600, .F. ) ;
#6854=CARTESIAN_POINT ( 'NONE',  ( 144.7991633467111683, 386.6211705227183870, 187.0000000000000568 ) ) ;
#6857=DIRECTION ( 'NONE',  ( -0.000000000000000000, -0.000000000000000000, 1.000000000000000000 ) ) ;
#6859=DIRECTION ( 'NONE',  ( -0.2873478855663477716, -0.9578262852211506528, 0.000000000000000000 ) ) ;
#6881=CARTESIAN_POINT ( 'NONE',  ( 610.8620436566991430, 230.3137853645740449, 190.0000000000000000 ) ) ;
#6909=DIRECTION ( 'NONE',  ( 0.000000000000000000, -1.000000000000000000, 0.000000000000000000 ) ) ;
#6946=VERTEX_POINT ( 'NONE', #1390 ) ;
#6977=DIRECTION ( 'NONE',  ( -0.9578262852211507639, 0.2873478855663477716, 0.000000000000000000 ) ) ;
#6990=EDGE_CURVE ( 'NONE', #7989, #3531, #3462, .T. ) ;
#7005=DIRECTION ( 'NONE',  ( 0.2873478855663503251, 0.9578262852211498757, 0.000000000000000000 ) ) ;
#7007=VECTOR ( 'NONE', #2413, 1000.000000000000000 ) ;
#7012=EDGE_CURVE ( 'NONE', #681, #8674, #11088, .T. ) ;
#7043=AXIS2_PLACEMENT_3D ( 'NONE', #7412, #8807, #3052 ) ;
#7046=AXIS2_PLACEMENT_3D ( 'NONE', #6426, #8701, #7229 ) ;
#7048=CARTESIAN_POINT ( 'NONE',  ( 611.4942090049449916, 232.4210031920597999, 184.7999999999999829 ) ) ;
#7049=LINE ( 'NONE', #250, #5651 ) ;
#7055=EDGE_LOOP ( 'NONE', ( #8356, #2793, #14278, #1756 ) ) ;
#7100=ORIENTED_EDGE ( 'NONE', *, *, #3002, .T. ) ;
#7101=AXIS2_PLACEMENT_3D ( 'NONE', #11138, #10854, #5254 ) ;
#7138=VERTEX_POINT ( 'NONE', #8908 ) ;
#7145=AXIS2_PLACEMENT_3D ( 'NONE', #4549, #2304, #6686 ) ;
#7153=ORIENTED_EDGE ( 'NONE', *, *, #561, .F. ) ;
#7205=( NAMED_UNIT ( * ) PLANE_ANGLE_UNIT ( ) SI_UNIT ( $, .RADIAN. ) );
#7209=EDGE_CURVE ( 'NONE', #2165, #2500, #5585, .T. ) ;
#7224=ORIENTED_EDGE ( 'NONE', *, *, #2833, .F. ) ;
#7229=DIRECTION ( 'NONE',  ( 0.000000000000000000, 1.000000000000000000, 3.264827003555234768E-15 ) ) ;
#7250=ORIENTED_EDGE ( 'NONE', *, *, #1504, .F. ) ;
#7265=CIRCLE ( 'NONE', #2549, 5.200000000000005507 ) ;
#7279=VECTOR ( 'NONE', #6859, 1000.000000000000000 ) ;
#7321=CIRCLE ( 'NONE', #9211, 4.199999999999926459 ) ;
#7322=CIRCLE ( 'NONE', #10858, 4.199999999999981526 ) ;
#7326=MECHANICAL_DESIGN_GEOMETRIC_PRESENTATION_REPRESENTATION('',(#3088),#953);
#7344=AXIS2_PLACEMENT_3D ( 'NONE', #1584, #10457, #11844 ) ;
#7354=DIRECTION ( 'NONE',  ( 0.9578262852211507639, -0.2873478855663477716, 0.000000000000000000 ) ) ;
#7364=DIRECTION ( 'NONE',  ( -1.000000000000000000, 0.000000000000000000, 0.000000000000000000 ) ) ;
#7386=DIRECTION ( 'NONE',  ( 0.2873478855663466613, 0.9578262852211509859, 0.000000000000000000 ) ) ;
#7391=CLOSED_SHELL ( 'NONE', ( #11467, #1131, #5423, #5132, #11065, #812, #10520, #1870, #2041, #5039, #11432, #6250, #1933, #6841, #3948, #3035, #7744, #9761, #160, #11055, #12050, #1374, #5142, #3920, #9451, #11294, #1044, #9174, #12211, #807 ) ) ;
#7412=CARTESIAN_POINT ( 'NONE',  ( 610.8620436566989156, 230.3137853645742155, -190.0000000000000000 ) ) ;
#7434=FACE_OUTER_BOUND ( 'NONE', #9587, .T. ) ;
#7480=EDGE_LOOP ( 'NONE', ( #2275, #7596, #2984, #3038 ) ) ;
#7521=FACE_BOUND ( 'NONE', #3298, .T. ) ;
#7531=DIRECTION ( 'NONE',  ( -0.000000000000000000, -0.000000000000000000, 1.000000000000000000 ) ) ;
#7543=CARTESIAN_POINT ( 'NONE',  ( 144.7991633467111683, 386.6211705227183870, -190.0000000000000568 ) ) ;
#7564=DIRECTION ( 'NONE',  ( 9.794481010665704304E-16, 3.264827003555233190E-15, 1.000000000000000000 ) ) ;
#7573=DIRECTION ( 'NONE',  ( 1.019665600948283644E-15, 3.398885336494278419E-15, -1.000000000000000000 ) ) ;
#7593=CARTESIAN_POINT ( 'NONE',  ( 153.1991633467111456, 386.6211705227183870, 210.0000000000000000 ) ) ;
#7596=ORIENTED_EDGE ( 'NONE', *, *, #14437, .T. ) ;
#7617=DIRECTION ( 'NONE',  ( 9.794481010665704304E-16, 3.264827003555233190E-15, 1.000000000000000000 ) ) ;
#7672=ORIENTED_EDGE ( 'NONE', *, *, #11012, .F. ) ;
#7691=DIRECTION ( 'NONE',  ( 1.460819769243627131E-16, 0.000000000000000000, -1.000000000000000000 ) ) ;
#7744=ADVANCED_FACE ( 'NONE', ( #824 ), #14276, .F. ) ;
#7749=FACE_OUTER_BOUND ( 'NONE', #6523, .T. ) ;
#7755=PRODUCT_CONTEXT ( 'NONE', #7830, 'mechanical' ) ;
#7760=DIRECTION ( 'NONE',  ( -9.223531621143024916E-30, 2.767059486342909086E-30, 1.000000000000000000 ) ) ;
#7770=CARTESIAN_POINT ( 'NONE',  ( 148.9991633467111569, 386.6211705227183870, 187.0000000000000568 ) ) ;
#7810=COLOUR_RGB ( '',0.8941176470588234615, 0.8941176470588234615, 0.8941176470588234615 ) ;
#7826=DIRECTION ( 'NONE',  ( -1.000802005371232860E-15, 0.000000000000000000, -1.000000000000000000 ) ) ;
#7830=APPLICATION_CONTEXT ( 'automotive_design' ) ;
#7855=CARTESIAN_POINT ( 'NONE',  ( -9.137956343300736251, 416.3137853645750397, -184.7999999999999829 ) ) ;
#7871=EDGE_LOOP ( 'NONE', ( #12347, #14170, #2149, #2274 ) ) ;
#7876=ORIENTED_EDGE ( 'NONE', *, *, #5314, .F. ) ;
#7898=DIRECTION ( 'NONE',  ( 0.2873478855663477161, 0.9578262852211506528, 0.000000000000000000 ) ) ;
#7906=DIRECTION ( 'NONE',  ( -0.2873478855663477161, -0.9578262852211506528, 0.000000000000000000 ) ) ;
#7939=VERTEX_POINT ( 'NONE', #1274 ) ;
#7942=DIRECTION ( 'NONE',  ( -7.885106708985460438E-16, 0.000000000000000000, -1.000000000000000000 ) ) ;
#7964=ORIENTED_EDGE ( 'NONE', *, *, #12675, .T. ) ;
#7967=AXIS2_PLACEMENT_3D ( 'NONE', #2913, #4101, #1648 ) ;
#7989=VERTEX_POINT ( 'NONE', #7855 ) ;
#8006=EDGE_CURVE ( 'NONE', #9048, #681, #2665, .T. ) ;
#8015=CARTESIAN_POINT ( 'NONE',  ( 611.4942090049451053, 232.4210031920598567, -190.0000000000000000 ) ) ;
#8024=ORIENTED_EDGE ( 'NONE', *, *, #2988, .T. ) ;
#8027=LINE ( 'NONE', #4641, #2320 ) ;
#8038=CARTESIAN_POINT ( 'NONE',  ( 610.0000000000001137, 227.4403065089106235, -184.8000000000000114 ) ) ;
#8039=ORIENTED_EDGE ( 'NONE', *, *, #2288, .T. ) ;
#8042=PLANE ( 'NONE',  #872 ) ;
#8095=ORIENTED_EDGE ( 'NONE', *, *, #1748, .F. ) ;
#8100=DIRECTION ( 'NONE',  ( -0.9578262852211513190, 0.2873478855663455511, -1.972152263052529951E-31 ) ) ;
#8131=EDGE_LOOP ( 'NONE', ( #11128, #8570, #13589, #8422 ) ) ;
#8186=DIRECTION ( 'NONE',  ( 4.427295178148650474E-30, -1.328188553444596088E-30, 1.000000000000000000 ) ) ;
#8203=AXIS2_PLACEMENT_3D ( 'NONE', #5535, #5470, #2960 ) ;
#8205=EDGE_CURVE ( 'NONE', #1376, #3502, #7322, .T. ) ;
#8236=ORIENTED_EDGE ( 'NONE', *, *, #8437, .T. ) ;
#8268=VERTEX_POINT ( 'NONE', #5178 ) ;
#8307=LINE ( 'NONE', #3893, #11119 ) ;
#8310=DIRECTION ( 'NONE',  ( 0.000000000000000000, 0.000000000000000000, 1.000000000000000000 ) ) ;
#8320=ORIENTED_EDGE ( 'NONE', *, *, #10968, .T. ) ;
#8337=CARTESIAN_POINT ( 'NONE',  ( 455.5035746174796714, 294.6698471414878782, -187.0000000000000568 ) ) ;
#8338=CARTESIAN_POINT ( 'NONE',  ( -8.505790995055004799, 418.4210031920606525, 190.0000000000000000 ) ) ;
#8348=ORIENTED_EDGE ( 'NONE', *, *, #8205, .T. ) ;
#8356=ORIENTED_EDGE ( 'NONE', *, *, #2027, .T. ) ;
#8378=DIRECTION ( 'NONE',  ( -0.000000000000000000, -0.000000000000000000, -1.000000000000000000 ) ) ;
#8422=ORIENTED_EDGE ( 'NONE', *, *, #1504, .T. ) ;
#8424=DIRECTION ( 'NONE',  ( -0.000000000000000000, -0.000000000000000000, -1.000000000000000000 ) ) ;
#8436=CIRCLE ( 'NONE', #2065, 4.199999999999981526 ) ;
#8437=EDGE_CURVE ( 'NONE', #3502, #1376, #4978, .T. ) ;
#8470=DIRECTION ( 'NONE',  ( -0.000000000000000000, -0.000000000000000000, -1.000000000000000000 ) ) ;
#8489=VECTOR ( 'NONE', #4155, 1000.000000000000227 ) ;
#8490=LINE ( 'NONE', #8338, #8619 ) ;
#8507=ORIENTED_EDGE ( 'NONE', *, *, #8993, .F. ) ;
#8508=( GEOMETRIC_REPRESENTATION_CONTEXT ( 3 ) GLOBAL_UNCERTAINTY_ASSIGNED_CONTEXT ( ( #6498 ) ) GLOBAL_UNIT_ASSIGNED_CONTEXT ( ( #6489, #3167, #2943 ) ) REPRESENTATION_CONTEXT ( 'NONE', 'WORKASPACE' ) );
#8515=CIRCLE ( 'NONE', #10402, 4.199999999999926459 ) ;
#8525=LINE ( 'NONE', #10809, #3790 ) ;
#8531=CARTESIAN_POINT ( 'NONE',  ( 611.4942090049448780, 232.4210031920607378, -190.0000000000000000 ) ) ;
#8538=AXIS2_PLACEMENT_3D ( 'NONE', #10026, #14532, #7826 ) ;
#8540=FACE_BOUND ( 'NONE', #1768, .T. ) ;
#8570=ORIENTED_EDGE ( 'NONE', *, *, #13921, .F. ) ;
#8587=LINE ( 'NONE', #6158, #14103 ) ;
#8593=ORIENTED_EDGE ( 'NONE', *, *, #1526, .F. ) ;
#8618=SURFACE_STYLE_FILL_AREA ( #10837 ) ;
#8619=VECTOR ( 'NONE', #8186, 1000.000000000000000 ) ;
#8661=EDGE_LOOP ( 'NONE', ( #8236, #8348 ) ) ;
#8674=VERTEX_POINT ( 'NONE', #14293 ) ;
#8693=VERTEX_POINT ( 'NONE', #2096 ) ;
#8697=AXIS2_PLACEMENT_3D ( 'NONE', #490, #12125, #10749 ) ;
#8701=DIRECTION ( 'NONE',  ( 9.794481010665704304E-16, 3.264827003555234768E-15, -1.000000000000000000 ) ) ;
#8711=LINE ( 'NONE', #8856, #9155 ) ;
#8737=VERTEX_POINT ( 'NONE', #9047 ) ;
#8768=AXIS2_PLACEMENT_3D ( 'NONE', #5970, #6255, #3909 ) ;
#8776=AXIS2_PLACEMENT_3D ( 'NONE', #9258, #533, #9400 ) ;
#8796=ORIENTED_EDGE ( 'NONE', *, *, #1966, .T. ) ;
#8807=DIRECTION ( 'NONE',  ( -0.9578262852211517631, 0.2873478855663442189, 4.622231866529365347E-30 ) ) ;
#8814=ORIENTED_EDGE ( 'NONE', *, *, #13790, .T. ) ;
#8824=CARTESIAN_POINT ( 'NONE',  ( 455.5035746174796714, 294.6698471414878782, -210.0000000000000000 ) ) ;
#8831=ORIENTED_EDGE ( 'NONE', *, *, #4768, .T. ) ;
#8845=CARTESIAN_POINT ( 'NONE',  ( 451.3035746174797396, 294.6698471414878782, -190.0000000000000568 ) ) ;
#8856=CARTESIAN_POINT ( 'NONE',  ( -8.505790995054995918, 418.4210031920607662, -187.0000000000000000 ) ) ;
#8866=CARTESIAN_POINT ( 'NONE',  ( 130.2060951089102332, 434.0203170297008910, 190.0000000000001990 ) ) ;
#8883=DIRECTION ( 'NONE',  ( -1.000000000000000000, 0.000000000000000000, 0.000000000000000000 ) ) ;
#8908=CARTESIAN_POINT ( 'NONE',  ( 451.3035746174797396, 294.6698471414878782, -187.0000000000000568 ) ) ;
#8911=ORIENTED_EDGE ( 'NONE', *, *, #6759, .T. ) ;
#8951=DIRECTION ( 'NONE',  ( -0.000000000000000000, -0.000000000000000000, 1.000000000000000000 ) ) ;
#8959=ORIENTED_EDGE ( 'NONE', *, *, #8006, .F. ) ;
#8993=EDGE_CURVE ( 'NONE', #2816, #1012, #1448, .T. ) ;
#9024=CARTESIAN_POINT ( 'NONE',  ( 7.240873133980779919, 470.9098836221796773, 187.0000000000001990 ) ) ;
#9047=CARTESIAN_POINT ( 'NONE',  ( 7.240873133980779919, 470.9098836221796773, 187.0000000000001990 ) ) ;
#9048=VERTEX_POINT ( 'NONE', #1796 ) ;
#9049=EDGE_CURVE ( 'NONE', #852, #8674, #10887, .T. ) ;
#9089=ORIENTED_EDGE ( 'NONE', *, *, #7209, .F. ) ;
#9096=EDGE_LOOP ( 'NONE', ( #12427, #7876, #14342, #5180 ) ) ;
#9097=CARTESIAN_POINT ( 'NONE',  ( 148.9991633467111569, 386.6211705227183870, -210.0000000000000000 ) ) ;
#9099=DIRECTION ( 'NONE',  ( 0.9578262852211507639, -0.2873478855663477716, -0.000000000000000000 ) ) ;
#9131=CARTESIAN_POINT ( 'NONE',  ( 611.4942090049448780, 232.4210031920607094, -187.0000000000000000 ) ) ;
#9155=VECTOR ( 'NONE', #868, 1000.000000000000000 ) ;
#9174=ADVANCED_FACE ( 'NONE', ( #3573 ), #12265, .F. ) ;
#9200=CARTESIAN_POINT ( 'NONE',  ( 153.1991633467111456, 386.6211705227183870, 187.0000000000000568 ) ) ;
#9211=AXIS2_PLACEMENT_3D ( 'NONE', #8337, #12776, #5101 ) ;
#9258=CARTESIAN_POINT ( 'NONE',  ( 7.240873133980776366, 470.9098836221796773, 190.0000000000001990 ) ) ;
#9277=PLANE ( 'NONE',  #4062 ) ;
#9284=EDGE_CURVE ( 'NONE', #13098, #5414, #1344, .T. ) ;
#9339=ORIENTED_EDGE ( 'NONE', *, *, #6263, .T. ) ;
#9365=CARTESIAN_POINT ( 'NONE',  ( -9.137956343300960071, 416.3137853645741302, 187.0000000000000000 ) ) ;
#9375=VECTOR ( 'NONE', #5004, 1000.000000000000000 ) ;
#9400=DIRECTION ( 'NONE',  ( 0.9578262852211513190, -0.2873478855663453846, 0.000000000000000000 ) ) ;
#9412=CARTESIAN_POINT ( 'NONE',  ( 144.7991633467111683, 386.6211705227183870, 210.0000000000000000 ) ) ;
#9416=DIRECTION ( 'NONE',  ( 9.963058866566173311E-16, 3.321019622188723911E-15, 1.000000000000000000 ) ) ;
#9427=ORIENTED_EDGE ( 'NONE', *, *, #4232, .T. ) ;
#9440=AXIS2_PLACEMENT_3D ( 'NONE', #4347, #14302, #6417 ) ;
#9451=ADVANCED_FACE ( 'NONE', ( #1633, #14047, #12929 ), #1718, .T. ) ;
#9504=STYLED_ITEM('',(#14660),#11971);
#9511=VECTOR ( 'NONE', #11839, 1000.000000000000000 ) ;
#9517=VERTEX_POINT ( 'NONE', #1777 ) ;
#9533=CARTESIAN_POINT ( 'NONE',  ( 455.5035746174796714, 294.6698471414878782, -210.0000000000000000 ) ) ;
#9561=EDGE_LOOP ( 'NONE', ( #1940, #2220, #8507, #5700 ) ) ;
#9587=EDGE_LOOP ( 'NONE', ( #14541, #8814, #14076, #3850 ) ) ;
#9593=FACE_OUTER_BOUND ( 'NONE', #7871, .T. ) ;
#9604=DIRECTION ( 'NONE',  ( 0.000000000000000000, -1.000000000000000000, 0.000000000000000000 ) ) ;
#9617=DIRECTION ( 'NONE',  ( 1.921916333308134107E-15, 6.406387777693825847E-15, -1.000000000000000000 ) ) ;
#9626=EDGE_CURVE ( 'NONE', #2500, #6946, #13655, .T. ) ;
#9633=VECTOR ( 'NONE', #6455, 1000.000000000000000 ) ;
#9693=CARTESIAN_POINT ( 'NONE',  ( -9.999999999999790390, 413.4403065089115330, -184.7999999999999829 ) ) ;
#9697=AXIS2_PLACEMENT_3D ( 'NONE', #9533, #1916, #1987 ) ;
#9704=PLANE ( 'NONE',  #7967 ) ;
#9724=CARTESIAN_POINT ( 'NONE',  ( 455.5035746174796714, 294.6698471414878782, 190.0000000000000568 ) ) ;
#9742=ORIENTED_EDGE ( 'NONE', *, *, #9626, .T. ) ;
#9746=VECTOR ( 'NONE', #1354, 1000.000000000000227 ) ;
#9750=PLANE ( 'NONE',  #12745 ) ;
#9755=LINE ( 'NONE', #3032, #379 ) ;
#9761=ADVANCED_FACE ( 'NONE', ( #4520 ), #13358, .T. ) ;
#9809=ORIENTED_EDGE ( 'NONE', *, *, #6446, .T. ) ;
#9811=EDGE_CURVE ( 'NONE', #12648, #2165, #220, .T. ) ;
#9814=CYLINDRICAL_SURFACE ( 'NONE', #9697, 4.199999999999926459 ) ;
#9818=LINE ( 'NONE', #5322, #862 ) ;
#9828=EDGE_CURVE ( 'NONE', #6153, #4085, #9830, .T. ) ;
#9830=LINE ( 'NONE', #8866, #8489 ) ;
#9846=DIRECTION ( 'NONE',  ( 0.2873478855663448850, 0.9578262852211515410, -3.408579461568462910E-15 ) ) ;
#9847=VECTOR ( 'NONE', #13178, 1000.000000000000227 ) ;
#9852=CARTESIAN_POINT ( 'NONE',  ( 130.2060951089103185, 434.0203170297010615, -190.0000000000001990 ) ) ;
#9870=CARTESIAN_POINT ( 'NONE',  ( 611.4942090049451053, 232.4210031920599420, -184.7999999999999829 ) ) ;
#9874=VERTEX_POINT ( 'NONE', #11222 ) ;
#9890=EDGE_CURVE ( 'NONE', #1912, #9874, #12111, .T. ) ;
#9904=AXIS2_PLACEMENT_3D ( 'NONE', #2007, #6522, #6459 ) ;
#9907=FACE_OUTER_BOUND ( 'NONE', #5760, .T. ) ;
#9923=PLANE ( 'NONE',  #8697 ) ;
#9956=EDGE_CURVE ( 'NONE', #12648, #7989, #3344, .T. ) ;
#9975=EDGE_LOOP ( 'NONE', ( #5790, #8831, #6663, #129 ) ) ;
#9984=CARTESIAN_POINT ( 'NONE',  ( 148.9991633467111569, 386.6211705227183870, -187.0000000000000568 ) ) ;
#10013=ORIENTED_EDGE ( 'NONE', *, *, #1858, .F. ) ;
#10023=DIRECTION ( 'NONE',  ( 9.794481010665704304E-16, 3.264827003555233190E-15, 1.000000000000000000 ) ) ;
#10026=CARTESIAN_POINT ( 'NONE',  ( -8.505790995054828940, 418.4210031920615620, -184.7999999999999829 ) ) ;
#10035=VERTEX_POINT ( 'NONE', #10200 ) ;
#10054=EDGE_CURVE ( 'NONE', #3531, #852, #2589, .T. ) ;
#10067=ORIENTED_EDGE ( 'NONE', *, *, #9956, .F. ) ;
#10080=CARTESIAN_POINT ( 'NONE',  ( -8.505790995054768544, 418.4210031920615620, -184.7999999999999829 ) ) ;
#10146=EDGE_CURVE ( 'NONE', #7138, #2902, #7321, .T. ) ;
#10184=CYLINDRICAL_SURFACE ( 'NONE', #1702, 4.199999999999981526 ) ;
#10200=CARTESIAN_POINT ( 'NONE',  ( 144.7991633467111683, 386.6211705227183870, -187.0000000000000568 ) ) ;
#10233=DIRECTION ( 'NONE',  ( -0.2873478855663503251, -0.9578262852211498757, 0.000000000000000000 ) ) ;
#10241=DIRECTION ( 'NONE',  ( 0.2873478855663478826, 0.9578262852211507639, 0.000000000000000000 ) ) ;
#10255=DIRECTION ( 'NONE',  ( 9.794481010665704304E-16, 3.264827003555234768E-15, -1.000000000000000000 ) ) ;
#10274=DIRECTION ( 'NONE',  ( -0.000000000000000000, -0.000000000000000000, 1.000000000000000000 ) ) ;
#10286=DIRECTION ( 'NONE',  ( 1.000000000000000000, 0.000000000000000000, 0.000000000000000000 ) ) ;
#10292=VERTEX_POINT ( 'NONE', #3026 ) ;
#10330=ORIENTED_EDGE ( 'NONE', *, *, #12621, .F. ) ;
#10363=CARTESIAN_POINT ( 'NONE',  ( 497.0347780250708638, -149.1104334075212421, -189.9999999999986358 ) ) ;
#10364=APPLICATION_CONTEXT ( 'automotive_design' ) ;
#10375=AXIS2_PLACEMENT_3D ( 'NONE', #11650, #1546, #7005 ) ;
#10398=CARTESIAN_POINT ( 'NONE',  ( 610.8620436566991430, 230.3137853645740449, 190.0000000000000000 ) ) ;
#10402=AXIS2_PLACEMENT_3D ( 'NONE', #1072, #12365, #3299 ) ;
#10406=CARTESIAN_POINT ( 'NONE',  ( -8.505790995054884007, 418.4210031920614483, 187.0000000000000000 ) ) ;
#10408=EDGE_LOOP ( 'NONE', ( #14161, #143, #571, #3050 ) ) ;
#10439=EDGE_CURVE ( 'NONE', #3223, #11084, #5924, .T. ) ;
#10447=VERTEX_POINT ( 'NONE', #5811 ) ;
#10457=DIRECTION ( 'NONE',  ( 0.9578262852211507639, -0.2873478855663477716, 0.000000000000000000 ) ) ;
#10480=VERTEX_POINT ( 'NONE', #6854 ) ;
#10511=EDGE_CURVE ( 'NONE', #13545, #10480, #2631, .T. ) ;
#10520=ADVANCED_FACE ( 'NONE', ( #4644 ), #2342, .T. ) ;
#10539=DIRECTION ( 'NONE',  ( -0.2873478855663466613, -0.9578262852211509859, -3.408579461568464883E-15 ) ) ;
#10572=EDGE_LOOP ( 'NONE', ( #7100, #14338, #11627, #14602 ) ) ;
#10628=EDGE_CURVE ( 'NONE', #1012, #2816, #245, .T. ) ;
#10655=EDGE_CURVE ( 'NONE', #9874, #2225, #789, .T. ) ;
#10662=CARTESIAN_POINT ( 'NONE',  ( 627.2408731339806991, 284.9098836221797342, 187.0000000000001990 ) ) ;
#10711=CARTESIAN_POINT ( 'NONE',  ( 610.8620436566991430, 230.3137853645733912, -184.7999999999999829 ) ) ;
#10719=CARTESIAN_POINT ( 'NONE',  ( -1.860589537588217608E-13, -6.201965125294058356E-13, 186.9999999999986358 ) ) ;
#10725=CARTESIAN_POINT ( 'NONE',  ( 611.4942090049448780, 232.4210031920607378, -189.9999999999999716 ) ) ;
#10744=FACE_OUTER_BOUND ( 'NONE', #13822, .T. ) ;
#10749=DIRECTION ( 'NONE',  ( 0.000000000000000000, -1.000000000000000000, 3.264827003555233190E-15 ) ) ;
#10808=EDGE_CURVE ( 'NONE', #13098, #4077, #8515, .T. ) ;
#10809=CARTESIAN_POINT ( 'NONE',  ( 7.240873133980834986, 470.9098836221799047, -187.0000000000001990 ) ) ;
#10818=DIRECTION ( 'NONE',  ( -0.2873478855663466613, -0.9578262852211509859, -3.408579461568464883E-15 ) ) ;
#10837=FILL_AREA_STYLE ('',( #6333 ) ) ;
#10845=ORIENTED_EDGE ( 'NONE', *, *, #10655, .T. ) ;
#10854=DIRECTION ( 'NONE',  ( 9.794481010665704304E-16, 3.264827003555234768E-15, -1.000000000000000000 ) ) ;
#10858=AXIS2_PLACEMENT_3D ( 'NONE', #12029, #7617, #9604 ) ;
#10859=DIRECTION ( 'NONE',  ( 0.9578262852211506528, -0.2873478855663477161, -0.000000000000000000 ) ) ;
#10865=ORIENTED_EDGE ( 'NONE', *, *, #14437, .F. ) ;
#10871=EDGE_CURVE ( 'NONE', #5524, #7989, #2154, .T. ) ;
#10887=LINE ( 'NONE', #13310, #5656 ) ;
#10953=DIRECTION ( 'NONE',  ( -0.000000000000000000, -0.000000000000000000, 1.000000000000000000 ) ) ;
#10968=EDGE_CURVE ( 'NONE', #2500, #681, #3351, .T. ) ;
#11005=AXIS2_PLACEMENT_3D ( 'NONE', #12654, #2406, #6909 ) ;
#11006=LINE ( 'NONE', #13159, #9633 ) ;
#11012=EDGE_CURVE ( 'NONE', #2902, #1012, #8307, .T. ) ;
#11017=DIRECTION ( 'NONE',  ( 0.000000000000000000, -1.000000000000000000, 0.000000000000000000 ) ) ;
#11019=AXIS2_PLACEMENT_3D ( 'NONE', #13430, #10255, #13734 ) ;
#11055=ADVANCED_FACE ( 'NONE', ( #5075 ), #11628, .T. ) ;
#11065=ADVANCED_FACE ( 'NONE', ( #12816 ), #9277, .F. ) ;
#11079=DIRECTION ( 'NONE',  ( 9.963058866566169367E-16, 3.321019622188723517E-15, 1.000000000000000000 ) ) ;
#11080=VECTOR ( 'NONE', #10274, 1000.000000000000000 ) ;
#11084=VERTEX_POINT ( 'NONE', #4036 ) ;
#11088=LINE ( 'NONE', #4811, #7279 ) ;
#11119=VECTOR ( 'NONE', #8378, 1000.000000000000000 ) ;
#11128=ORIENTED_EDGE ( 'NONE', *, *, #12621, .T. ) ;
#11138=CARTESIAN_POINT ( 'NONE',  ( 148.9991633467111569, 386.6211705227183870, 190.0000000000000568 ) ) ;
#11176=ORIENTED_EDGE ( 'NONE', *, *, #7012, .F. ) ;
#11202=CARTESIAN_POINT ( 'NONE',  ( 459.7035746174795463, 294.6698471414878782, 187.0000000000000568 ) ) ;
#11219=CARTESIAN_POINT ( 'NONE',  ( -8.505790995054884007, 418.4210031920614483, 184.7999999999999829 ) ) ;
#11222=CARTESIAN_POINT ( 'NONE',  ( 627.2408731339805854, 284.9098836221799615, -187.0000000000001990 ) ) ;
#11228=LINE ( 'NONE', #9024, #14115 ) ;
#11240=EDGE_LOOP ( 'NONE', ( #13092, #8911, #7250, #8095 ) ) ;
#11280=DIRECTION ( 'NONE',  ( -0.9578262852211506528, 0.2873478855663477161, -0.000000000000000000 ) ) ;
#11294=ADVANCED_FACE ( 'NONE', ( #12575 ), #5937, .F. ) ;
#11302=CARTESIAN_POINT ( 'NONE',  ( -9.137956343300835726, 416.3137853645748692, 184.7999999999999829 ) ) ;
#11377=MECHANICAL_DESIGN_GEOMETRIC_PRESENTATION_REPRESENTATION('',(#9504),#2424);
#11396=DIRECTION ( 'NONE',  ( 0.9578262852211507639, -0.2873478855663477716, -0.000000000000000000 ) ) ;
#11427=CARTESIAN_POINT ( 'NONE',  ( -9.137956343300736251, 416.3137853645750397, -184.7999999999999829 ) ) ;
#11432=ADVANCED_FACE ( 'NONE', ( #2201 ), #6566, .T. ) ;
#11435=EDGE_LOOP ( 'NONE', ( #10865, #7224, #985, #605 ) ) ;
#11459=FACE_OUTER_BOUND ( 'NONE', #7055, .T. ) ;
#11467=ADVANCED_FACE ( 'NONE', ( #1384 ), #10184, .F. ) ;
#11482=CARTESIAN_POINT ( 'NONE',  ( 459.7035746174795463, 294.6698471414878782, -187.0000000000000568 ) ) ;
#11510=DIRECTION ( 'NONE',  ( 0.9578262852211506528, -0.2873478855663477161, -0.000000000000000000 ) ) ;
#11563=FACE_BOUND ( 'NONE', #100, .T. ) ;
#11567=AXIS2_PLACEMENT_3D ( 'NONE', #429, #9099, #3422 ) ;
#11572=AXIS2_PLACEMENT_3D ( 'NONE', #10398, #4726, #2428 ) ;
#11627=ORIENTED_EDGE ( 'NONE', *, *, #6446, .F. ) ;
#11628=CYLINDRICAL_SURFACE ( 'NONE', #12773, 5.200000000000009948 ) ;
#11650=CARTESIAN_POINT ( 'NONE',  ( -8.505790995054884007, 418.4210031920614483, 184.7999999999999829 ) ) ;
#11682=ORIENTED_EDGE ( 'NONE', *, *, #8993, .T. ) ;
#11702=ORIENTED_EDGE ( 'NONE', *, *, #11840, .F. ) ;
#11714=ORIENTED_EDGE ( 'NONE', *, *, #10808, .T. ) ;
#11764=EDGE_CURVE ( 'NONE', #13545, #11084, #4346, .T. ) ;
#11826=LINE ( 'NONE', #10725, #12561 ) ;
#11839=DIRECTION ( 'NONE',  ( -0.000000000000000000, -0.000000000000000000, 1.000000000000000000 ) ) ;
#11840=EDGE_CURVE ( 'NONE', #9048, #2225, #12793, .T. ) ;
#11844=DIRECTION ( 'NONE',  ( 0.2873478855663396114, 0.9578262852211530953, 0.000000000000000000 ) ) ;
#11845=CARTESIAN_POINT ( 'NONE',  ( 7.240873133980776366, 470.9098836221796773, 190.0000000000001990 ) ) ;
#11881=DIRECTION ( 'NONE',  ( 0.2873478855663427756, 0.9578262852211522071, 3.408579461568464094E-15 ) ) ;
#11929=ORIENTED_EDGE ( 'NONE', *, *, #6263, .F. ) ;
#11933=FACE_OUTER_BOUND ( 'NONE', #9561, .T. ) ;
#11936=PRODUCT ( 'stationary channel', 'stationary channel', '', ( #7755 ) ) ;
#11971=MANIFOLD_SOLID_BREP ( 'Mirror2', #7391 ) ;
#11972=ORIENTED_EDGE ( 'NONE', *, *, #1375, .F. ) ;
#11976=CIRCLE ( 'NONE', #3270, 4.199999999999981526 ) ;
#11992=DIRECTION ( 'NONE',  ( 0.000000000000000000, 1.000000000000000000, 0.000000000000000000 ) ) ;
#11997=VECTOR ( 'NONE', #5827, 1000.000000000000000 ) ;
#12000=CARTESIAN_POINT ( 'NONE',  ( 148.9991633467111569, 386.6211705227183870, -210.0000000000000000 ) ) ;
#12004=VECTOR ( 'NONE', #14598, 1000.000000000000000 ) ;
#12029=CARTESIAN_POINT ( 'NONE',  ( 148.9991633467111569, 386.6211705227183870, -190.0000000000000568 ) ) ;
#12050=ADVANCED_FACE ( 'NONE', ( #10744 ), #2852, .F. ) ;
#12109=EDGE_CURVE ( 'NONE', #14129, #10035, #5485, .T. ) ;
#12111=LINE ( 'NONE', #13152, #233 ) ;
#12125=DIRECTION ( 'NONE',  ( 9.794481010665704304E-16, 3.264827003555233190E-15, 1.000000000000000000 ) ) ;
#12167=CARTESIAN_POINT ( 'NONE',  ( 148.9991633467111569, 386.6211705227183870, -190.0000000000000568 ) ) ;
#12173=EDGE_CURVE ( 'NONE', #1912, #13547, #1961, .T. ) ;
#12207=CIRCLE ( 'NONE', #1141, 5.200000000000004619 ) ;
#12211=ADVANCED_FACE ( 'NONE', ( #3588 ), #5566, .F. ) ;
#12214=( NAMED_UNIT ( * ) PLANE_ANGLE_UNIT ( ) SI_UNIT ( $, .RADIAN. ) );
#12238=SHAPE_DEFINITION_REPRESENTATION ( #2505, #2248 ) ;
#12258=DIRECTION ( 'NONE',  ( 9.794481010665704304E-16, 3.264827003555234768E-15, -1.000000000000000000 ) ) ;
#12259=CARTESIAN_POINT ( 'NONE',  ( 148.9991633467111569, 386.6211705227183870, 190.0000000000000568 ) ) ;
#12265=CYLINDRICAL_SURFACE ( 'NONE', #2143, 4.199999999999981526 ) ;
#12280=EDGE_LOOP ( 'NONE', ( #3276, #14589, #14088, #4367 ) ) ;
#12347=ORIENTED_EDGE ( 'NONE', *, *, #561, .T. ) ;
#12365=DIRECTION ( 'NONE',  ( 9.794481010665704304E-16, 3.264827003555234768E-15, -1.000000000000000000 ) ) ;
#12381=LINE ( 'NONE', #108, #5665 ) ;
#12389=ORIENTED_EDGE ( 'NONE', *, *, #2288, .F. ) ;
#12427=ORIENTED_EDGE ( 'NONE', *, *, #4847, .F. ) ;
#12437=LINE ( 'NONE', #2325, #7007 ) ;
#12443=EDGE_LOOP ( 'NONE', ( #4675, #8959, #2661, #10067 ) ) ;
#12451=DIRECTION ( 'NONE',  ( 1.000000000000000000, 0.000000000000000000, 0.000000000000000000 ) ) ;
#12490=ORIENTED_EDGE ( 'NONE', *, *, #9956, .T. ) ;
#12508=VECTOR ( 'NONE', #8100, 1000.000000000000114 ) ;
#12512=AXIS2_PLACEMENT_3D ( 'NONE', #3619, #4577, #12607 ) ;
#12520=ADVANCED_BREP_SHAPE_REPRESENTATION ( '', ( #11971, #9440 ), #8508 ) ;
#12535=AXIS2_PLACEMENT_3D ( 'NONE', #10080, #6977, #10233 ) ;
#12558=AXIS2_PLACEMENT_3D ( 'NONE', #9870, #5521, #2107 ) ;
#12560=ORIENTED_EDGE ( 'NONE', *, *, #9811, .T. ) ;
#12561=VECTOR ( 'NONE', #9617, 1000.000000000000000 ) ;
#12575=FACE_OUTER_BOUND ( 'NONE', #8131, .T. ) ;
#12597=AXIS2_PLACEMENT_3D ( 'NONE', #13428, #6857, #12451 ) ;
#12607=DIRECTION ( 'NONE',  ( 0.000000000000000000, 1.000000000000000000, 0.000000000000000000 ) ) ;
#12621=EDGE_CURVE ( 'NONE', #7939, #8737, #11228, .T. ) ;
#12648=VERTEX_POINT ( 'NONE', #11302 ) ;
#12654=CARTESIAN_POINT ( 'NONE',  ( 455.5035746174796714, 294.6698471414878782, -187.0000000000000568 ) ) ;
#12666=ORIENTED_EDGE ( 'NONE', *, *, #6401, .T. ) ;
#12675=EDGE_CURVE ( 'NONE', #11084, #3223, #11976, .T. ) ;
#12678=LINE ( 'NONE', #9365, #14252 ) ;
#12684=ORIENTED_EDGE ( 'NONE', *, *, #3700, .F. ) ;
#12704=CIRCLE ( 'NONE', #5168, 4.199999999999926459 ) ;
#12721=CARTESIAN_POINT ( 'NONE',  ( 611.4942090049451053, 232.4210031920599135, -184.7999999999999829 ) ) ;
#12726=ORIENTED_EDGE ( 'NONE', *, *, #9811, .F. ) ;
#12745=AXIS2_PLACEMENT_3D ( 'NONE', #6428, #576, #7386 ) ;
#12773=AXIS2_PLACEMENT_3D ( 'NONE', #7048, #249, #3955 ) ;
#12776=DIRECTION ( 'NONE',  ( -9.794481010665704304E-16, -3.264827003555233190E-15, -1.000000000000000000 ) ) ;
#12789=DIRECTION ( 'NONE',  ( 9.794481010665704304E-16, 3.264827003555233190E-15, 1.000000000000000000 ) ) ;
#12793=CIRCLE ( 'NONE', #12558, 2.200000000000009948 ) ;
#12800=CARTESIAN_POINT ( 'NONE',  ( 153.1991633467111456, 386.6211705227183870, -187.0000000000000568 ) ) ;
#12816=FACE_OUTER_BOUND ( 'NONE', #12443, .T. ) ;
#12852=LINE ( 'NONE', #2672, #3506 ) ;
#12864=CARTESIAN_POINT ( 'NONE',  ( 451.3035746174797396, 294.6698471414878782, -210.0000000000000000 ) ) ;
#12900=VECTOR ( 'NONE', #3924, 999.9999999999998863 ) ;
#12915=PLANE ( 'NONE',  #7046 ) ;
#12929=FACE_OUTER_BOUND ( 'NONE', #13468, .T. ) ;
#12936=ORIENTED_EDGE ( 'NONE', *, *, #13790, .F. ) ;
#12937=DIRECTION ( 'NONE',  ( -0.9578262852211507639, 0.2873478855663477716, 0.000000000000000000 ) ) ;
#12971=FACE_OUTER_BOUND ( 'NONE', #9096, .T. ) ;
#13023=DIRECTION ( 'NONE',  ( 0.000000000000000000, 1.000000000000000000, 0.000000000000000000 ) ) ;
#13059=CARTESIAN_POINT ( 'NONE',  ( -8.505790995054992365, 418.4210031920607662, -190.0000000000000000 ) ) ;
#13061=ORIENTED_EDGE ( 'NONE', *, *, #1748, .T. ) ;
#13092=ORIENTED_EDGE ( 'NONE', *, *, #9626, .F. ) ;
#13098=VERTEX_POINT ( 'NONE', #3626 ) ;
#13122=SURFACE_SIDE_STYLE ('',( #8618 ) ) ;
#13139=ORIENTED_EDGE ( 'NONE', *, *, #4768, .F. ) ;
#13141=FACE_OUTER_BOUND ( 'NONE', #1176, .T. ) ;
#13152=CARTESIAN_POINT ( 'NONE',  ( 627.2408731339805854, 284.9098836221799615, -190.0000000000001990 ) ) ;
#13159=CARTESIAN_POINT ( 'NONE',  ( 627.2408731339806991, 284.9098836221797342, 190.0000000000001990 ) ) ;
#13178=DIRECTION ( 'NONE',  ( 0.9578262852211513190, -0.2873478855663454401, -1.972152263052529514E-31 ) ) ;
#13183=EDGE_LOOP ( 'NONE', ( #11972, #13061, #5152, #12666 ) ) ;
#13199=VECTOR ( 'NONE', #7573, 1000.000000000000000 ) ;
#13216=AXIS2_PLACEMENT_3D ( 'NONE', #12167, #12789, #2055 ) ;
#13247=EDGE_CURVE ( 'NONE', #5414, #8268, #679, .T. ) ;
#13260=DIRECTION ( 'NONE',  ( -9.794481010665704304E-16, -3.264827003555233190E-15, -1.000000000000000000 ) ) ;
#13310=CARTESIAN_POINT ( 'NONE',  ( 610.0000000000001137, 227.4403065089106235, 190.0000000000000000 ) ) ;
#13321=LINE ( 'NONE', #9852, #9847 ) ;
#13344=FACE_OUTER_BOUND ( 'NONE', #1869, .T. ) ;
#13355=ORIENTED_EDGE ( 'NONE', *, *, #6759, .F. ) ;
#13358=PLANE ( 'NONE',  #6383 ) ;
#13383=ORIENTED_EDGE ( 'NONE', *, *, #2833, .T. ) ;
#13419=CARTESIAN_POINT ( 'NONE',  ( -1.891202423064421949E-13, -6.304008076881404142E-13, -189.9999999999986358 ) ) ;
#13427=CARTESIAN_POINT ( 'NONE',  ( 144.7991633467111683, 386.6211705227183870, -210.0000000000000000 ) ) ;
#13428=CARTESIAN_POINT ( 'NONE',  ( 148.9991633467111569, 386.6211705227183870, 210.0000000000000000 ) ) ;
#13430=CARTESIAN_POINT ( 'NONE',  ( 455.5035746174796714, 294.6698471414878782, 187.0000000000000568 ) ) ;
#13443=AXIS2_PLACEMENT_3D ( 'NONE', #10719, #588, #958 ) ;
#13447=UNCERTAINTY_MEASURE_WITH_UNIT (LENGTH_MEASURE( 1.000000000000000082E-05 ), #2705, 'distance_accuracy_value', 'NONE');
#13457=EDGE_LOOP ( 'NONE', ( #5848, #8593 ) ) ;
#13468=EDGE_LOOP ( 'NONE', ( #13355, #9089, #4815, #10330 ) ) ;
#13510=VERTEX_POINT ( 'NONE', #13059 ) ;
#13545=VERTEX_POINT ( 'NONE', #9200 ) ;
#13547=VERTEX_POINT ( 'NONE', #8015 ) ;
#13589=ORIENTED_EDGE ( 'NONE', *, *, #9828, .F. ) ;
#13591=DIRECTION ( 'NONE',  ( -0.9578262852211513190, 0.2873478855663453846, -0.000000000000000000 ) ) ;
#13632=DIRECTION ( 'NONE',  ( 0.9578262852211513190, -0.2873478855663454401, -1.972152263052529514E-31 ) ) ;
#13633=AXIS2_PLACEMENT_3D ( 'NONE', #3233, #1014, #858 ) ;
#13655=LINE ( 'NONE', #1178, #1423 ) ;
#13734=DIRECTION ( 'NONE',  ( 0.000000000000000000, 1.000000000000000000, 0.000000000000000000 ) ) ;
#13736=ORIENTED_EDGE ( 'NONE', *, *, #6407, .T. ) ;
#13779=CARTESIAN_POINT ( 'NONE',  ( 113.8272656316285776, 379.4242187720952870, 1.650218294979717018E-14 ) ) ;
#13790=EDGE_CURVE ( 'NONE', #14129, #1376, #7049, .T. ) ;
#13822=EDGE_LOOP ( 'NONE', ( #9427, #12560, #4396, #8320 ) ) ;
#13828=CARTESIAN_POINT ( 'NONE',  ( 455.5035746174796714, 294.6698471414878782, 210.0000000000000000 ) ) ;
#13845=( NAMED_UNIT ( * ) SI_UNIT ( $, .STERADIAN. ) SOLID_ANGLE_UNIT ( ) );
#13857=LINE ( 'NONE', #9131, #12508 ) ;
#13876=ORIENTED_EDGE ( 'NONE', *, *, #1901, .T. ) ;
#13921=EDGE_CURVE ( 'NONE', #4085, #8737, #1802, .T. ) ;
#13957=ORIENTED_EDGE ( 'NONE', *, *, #10871, .T. ) ;
#13981=PRODUCT_DEFINITION_FORMATION_WITH_SPECIFIED_SOURCE ( 'ANY', '', #11936, .NOT_KNOWN. ) ;
#14047=FACE_BOUND ( 'NONE', #4669, .T. ) ;
#14076=ORIENTED_EDGE ( 'NONE', *, *, #8437, .F. ) ;
#14088=ORIENTED_EDGE ( 'NONE', *, *, #9049, .F. ) ;
#14103=VECTOR ( 'NONE', #535, 1000.000000000000000 ) ;
#14115=VECTOR ( 'NONE', #13591, 1000.000000000000227 ) ;
#14129=VERTEX_POINT ( 'NONE', #12800 ) ;
#14161=ORIENTED_EDGE ( 'NONE', *, *, #10871, .F. ) ;
#14170=ORIENTED_EDGE ( 'NONE', *, *, #6401, .F. ) ;
#14172=ORIENTED_EDGE ( 'NONE', *, *, #4847, .T. ) ;
#14186=CARTESIAN_POINT ( 'NONE',  ( 7.240873133980832321, 470.9098836221799047, -190.0000000000001990 ) ) ;
#14214=ORIENTED_EDGE ( 'NONE', *, *, #13247, .T. ) ;
#14252=VECTOR ( 'NONE', #10539, 1000.000000000000114 ) ;
#14256=PLANE ( 'NONE',  #6058 ) ;
#14276=PLANE ( 'NONE',  #9904 ) ;
#14278=ORIENTED_EDGE ( 'NONE', *, *, #6816, .F. ) ;
#14284=EDGE_LOOP ( 'NONE', ( #5946, #1373, #13736, #628 ) ) ;
#14293=CARTESIAN_POINT ( 'NONE',  ( 609.9999999999998863, 227.4403065089098277, 184.7999999999999829 ) ) ;
#14302=DIRECTION ( 'NONE',  ( 0.000000000000000000, 0.000000000000000000, 1.000000000000000000 ) ) ;
#14304=EDGE_CURVE ( 'NONE', #10035, #3502, #2827, .T. ) ;
#14338=ORIENTED_EDGE ( 'NONE', *, *, #9890, .F. ) ;
#14342=ORIENTED_EDGE ( 'NONE', *, *, #10655, .F. ) ;
#14387=CARTESIAN_POINT ( 'NONE',  ( 7.240873133980792353, 470.9098836221797342, 190.0000000000001990 ) ) ;
#14396=CARTESIAN_POINT ( 'NONE',  ( 627.2408731339806991, 284.9098836221800184, -190.0000000000001990 ) ) ;
#14420=FACE_OUTER_BOUND ( 'NONE', #4380, .T. ) ;
#14437=EDGE_CURVE ( 'NONE', #8674, #9517, #12381, .T. ) ;
#14460=ORIENTED_EDGE ( 'NONE', *, *, #10146, .F. ) ;
#14477=ORIENTED_EDGE ( 'NONE', *, *, #1726, .T. ) ;
#14502=CYLINDRICAL_SURFACE ( 'NONE', #4203, 4.199999999999926459 ) ;
#14532=DIRECTION ( 'NONE',  ( -0.9578262852211507639, 0.2873478855663477716, 0.000000000000000000 ) ) ;
#14541=ORIENTED_EDGE ( 'NONE', *, *, #12109, .F. ) ;
#14548=ORIENTED_EDGE ( 'NONE', *, *, #5847, .T. ) ;
#14566=EDGE_LOOP ( 'NONE', ( #5510, #11702, #14477, #6299 ) ) ;
#14589=ORIENTED_EDGE ( 'NONE', *, *, #7012, .T. ) ;
#14594=CARTESIAN_POINT ( 'NONE',  ( -8.505790995054828940, 418.4210031920615620, -184.7999999999999829 ) ) ;
#14598=DIRECTION ( 'NONE',  ( 0.9578262852211513190, -0.2873478855663455511, -5.916456789157588541E-31 ) ) ;
#14602=ORIENTED_EDGE ( 'NONE', *, *, #2307, .T. ) ;
#14610=VECTOR ( 'NONE', #626, 1000.000000000000114 ) ;
#14614=CYLINDRICAL_SURFACE ( 'NONE', #12597, 4.199999999999981526 ) ;
#14654=COLOUR_RGB('Light Blue',0.38,0.62,0.78);
#14655=FILL_AREA_STYLE_COLOUR('',#14654);
#14656=FILL_AREA_STYLE('',(#14655));
#14657=SURFACE_STYLE_FILL_AREA(#14656);
#14658=SURFACE_SIDE_STYLE('',(#14657));
#14659=SURFACE_STYLE_USAGE(.BOTH.,#14658);
#14660=PRESENTATION_STYLE_ASSIGNMENT((#14659));
ENDSEC;
END-ISO-10303-21;
